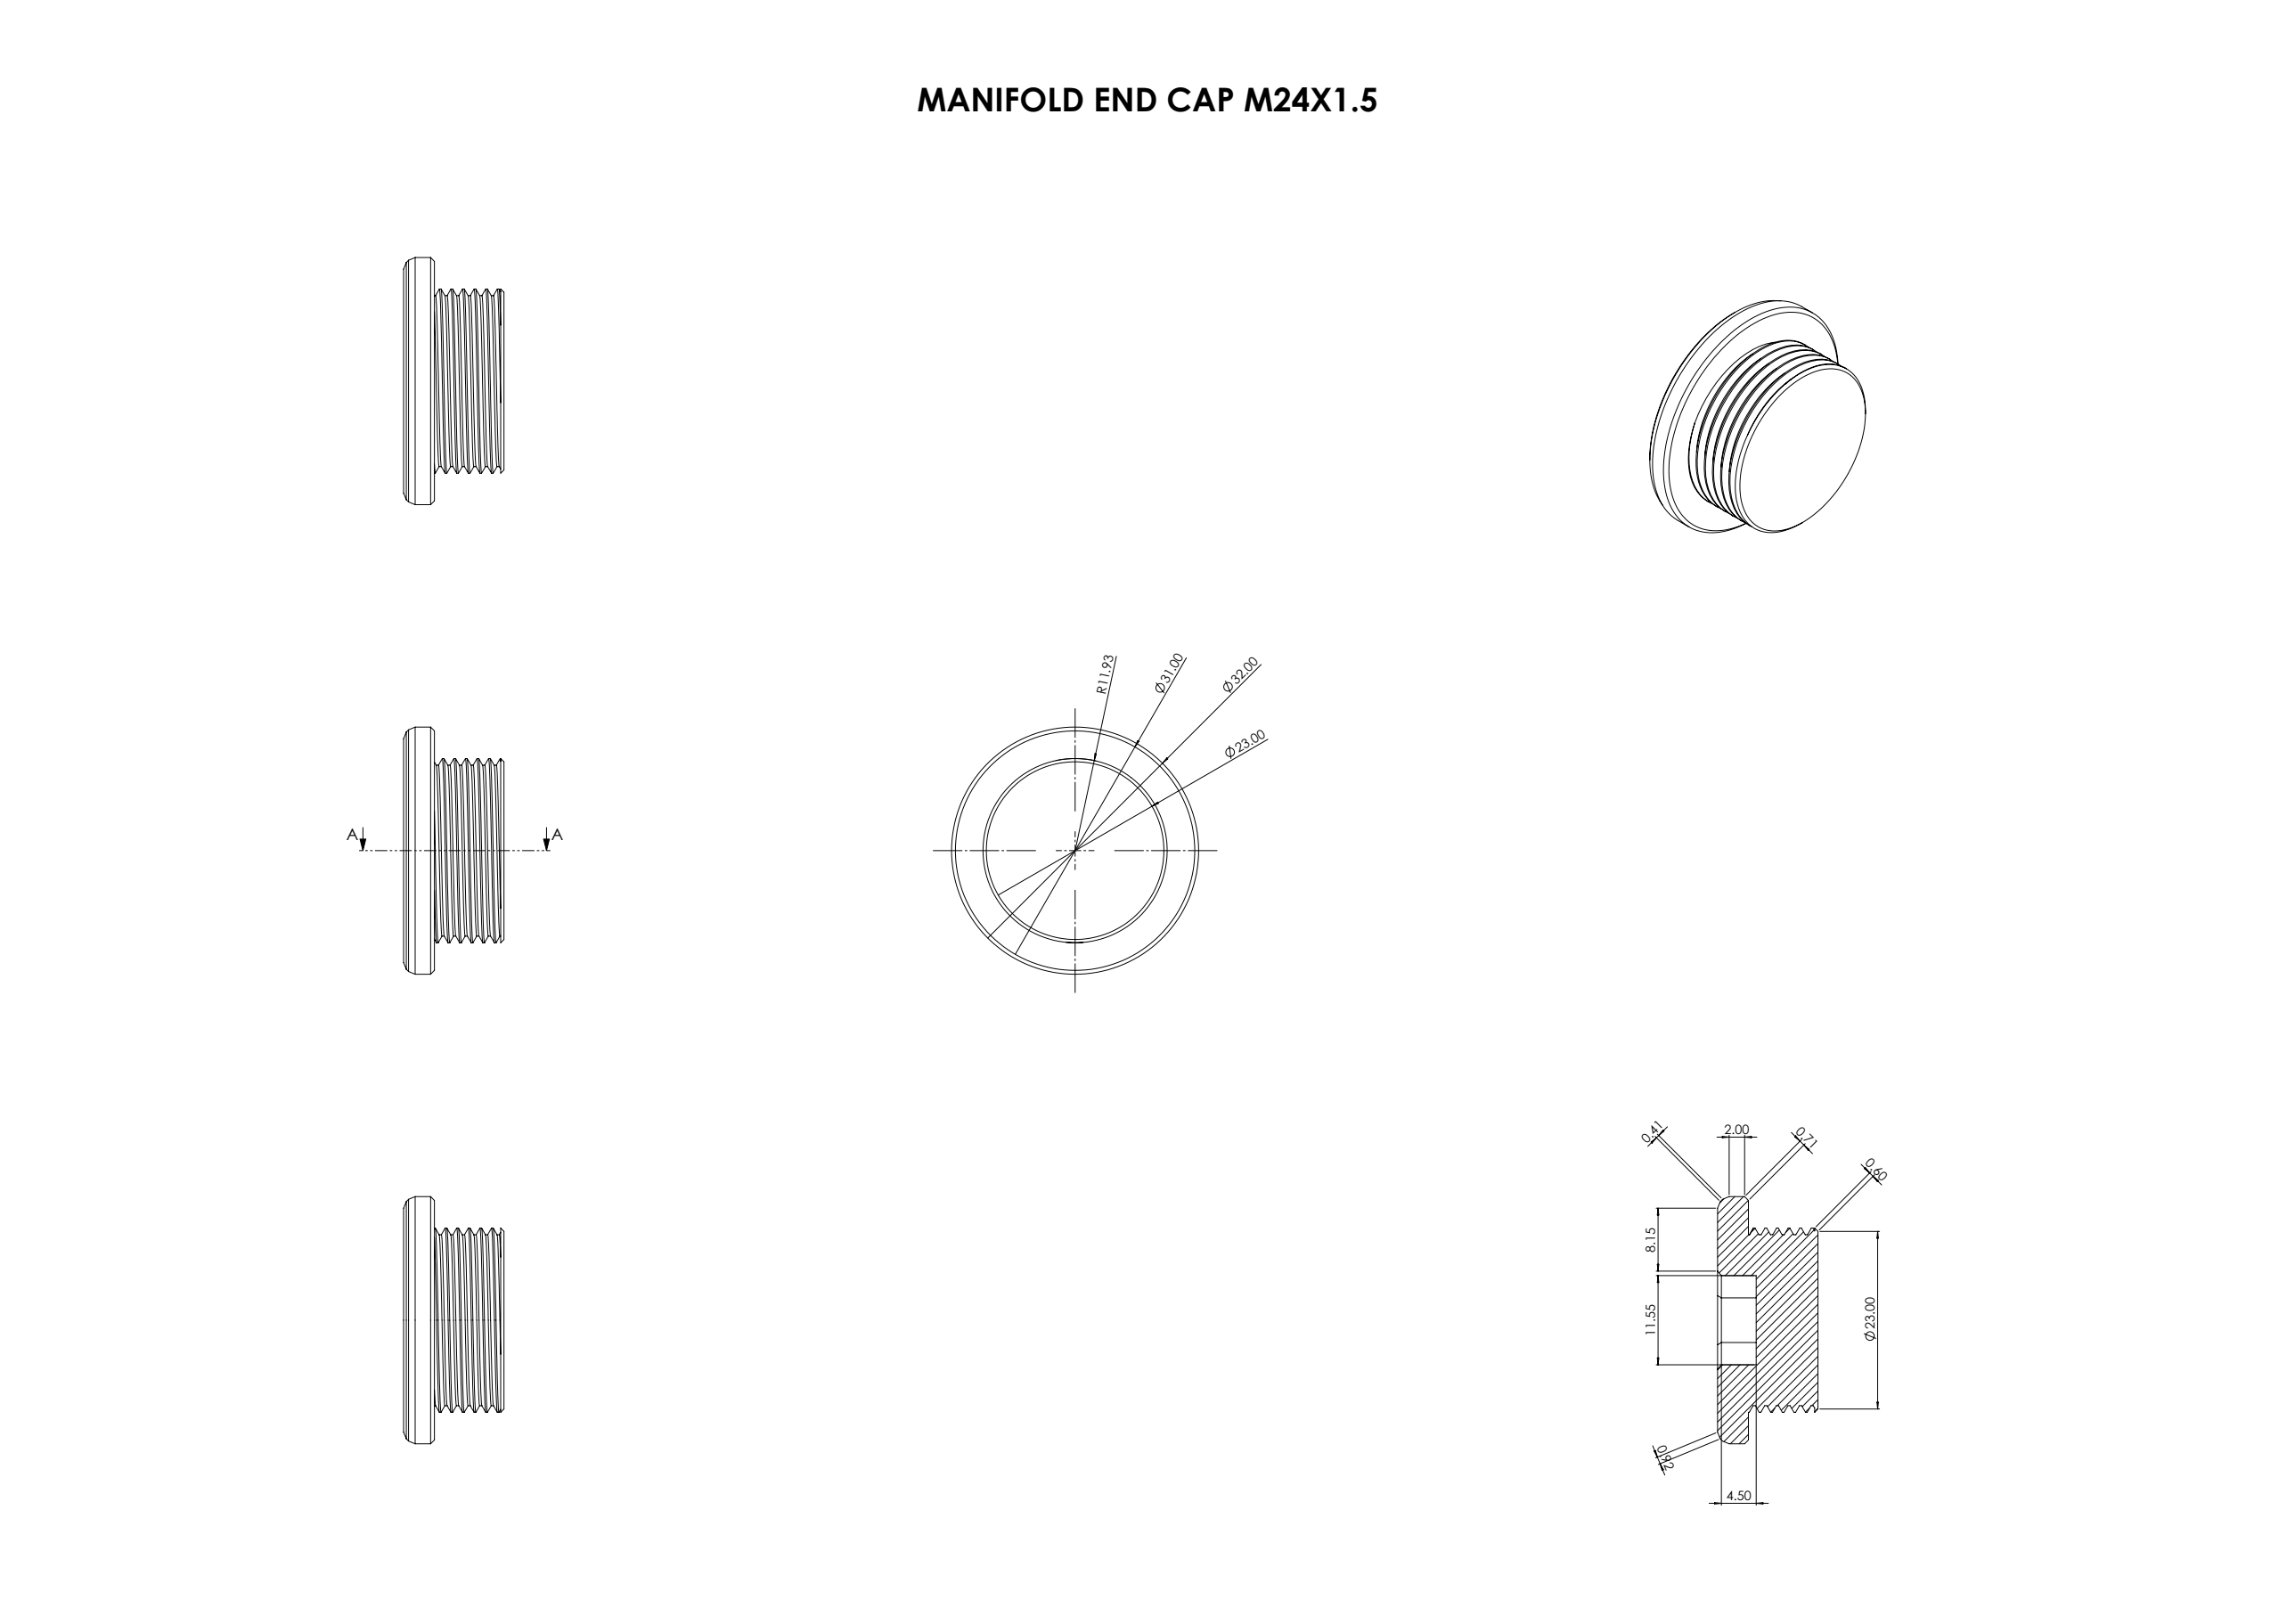
ISO-10303-21;
HEADER;
/* Generated by software containing ST-Developer
 * from STEP Tools, Inc. (www.steptools.com) 
 */

FILE_DESCRIPTION(
/* description */ (''),
/* implementation_level */ '2;1');

FILE_NAME(
/* name */ '11_Manifold_End_Cap_M24x1.5.step',
/* time_stamp */ '2026-10-26T06:13:19-07:00',
/* author */ (''),
/* organization */ (''),
/* preprocessor_version */ 'ST-DEVELOPER v20.2',
/* originating_system */ 'Autodesk Translation Framework v15.15.0.0',
/* authorisation */ '');

FILE_SCHEMA (('AUTOMOTIVE_DESIGN { 1 0 10303 214 3 1 1 }','TECHNICAL_DATA_PACKAGING'));
ENDSEC;

DATA;
#10=MECHANICAL_DESIGN_GEOMETRIC_PRESENTATION_REPRESENTATION('',(#307),#56639);
#267=SHAPE_REPRESENTATION_RELATIONSHIP('SRR','None',#56755,#287);
#287=ADVANCED_BREP_SHAPE_REPRESENTATION('',(#327),#56629);
#307=STYLED_ITEM('',(#56901),#327);
#327=MANIFOLD_SOLID_BREP('Body1',#16959);
#353=B_SPLINE_SURFACE_WITH_KNOTS('',3,3,((#35356,#35357,#35358,#35359,#35360,
#35361,#35362,#35363,#35364,#35365,#35366,#35367,#35368,#35369,#35370,#35371,
#35372,#35373,#35374,#35375,#35376,#35377,#35378,#35379,#35380,#35381,#35382,
#35383,#35384,#35385,#35386,#35387,#35388,#35389,#35390,#35391,#35392,#35393,
#35394,#35395,#35396,#35397,#35398,#35399,#35400,#35401,#35402,#35403,#35404,
#35405,#35406,#35407,#35408,#35409,#35410,#35411,#35412,#35413,#35414,#35415,
#35416,#35417,#35418,#35419,#35420,#35421,#35422,#35423,#35424,#35425,#35426,
#35427,#35428,#35429,#35430,#35431,#35432,#35433,#35434),(#35435,#35436,
#35437,#35438,#35439,#35440,#35441,#35442,#35443,#35444,#35445,#35446,#35447,
#35448,#35449,#35450,#35451,#35452,#35453,#35454,#35455,#35456,#35457,#35458,
#35459,#35460,#35461,#35462,#35463,#35464,#35465,#35466,#35467,#35468,#35469,
#35470,#35471,#35472,#35473,#35474,#35475,#35476,#35477,#35478,#35479,#35480,
#35481,#35482,#35483,#35484,#35485,#35486,#35487,#35488,#35489,#35490,#35491,
#35492,#35493,#35494,#35495,#35496,#35497,#35498,#35499,#35500,#35501,#35502,
#35503,#35504,#35505,#35506,#35507,#35508,#35509,#35510,#35511,#35512,#35513),
(#35514,#35515,#35516,#35517,#35518,#35519,#35520,#35521,#35522,#35523,
#35524,#35525,#35526,#35527,#35528,#35529,#35530,#35531,#35532,#35533,#35534,
#35535,#35536,#35537,#35538,#35539,#35540,#35541,#35542,#35543,#35544,#35545,
#35546,#35547,#35548,#35549,#35550,#35551,#35552,#35553,#35554,#35555,#35556,
#35557,#35558,#35559,#35560,#35561,#35562,#35563,#35564,#35565,#35566,#35567,
#35568,#35569,#35570,#35571,#35572,#35573,#35574,#35575,#35576,#35577,#35578,
#35579,#35580,#35581,#35582,#35583,#35584,#35585,#35586,#35587,#35588,#35589,
#35590,#35591,#35592),(#35593,#35594,#35595,#35596,#35597,#35598,#35599,
#35600,#35601,#35602,#35603,#35604,#35605,#35606,#35607,#35608,#35609,#35610,
#35611,#35612,#35613,#35614,#35615,#35616,#35617,#35618,#35619,#35620,#35621,
#35622,#35623,#35624,#35625,#35626,#35627,#35628,#35629,#35630,#35631,#35632,
#35633,#35634,#35635,#35636,#35637,#35638,#35639,#35640,#35641,#35642,#35643,
#35644,#35645,#35646,#35647,#35648,#35649,#35650,#35651,#35652,#35653,#35654,
#35655,#35656,#35657,#35658,#35659,#35660,#35661,#35662,#35663,#35664,#35665,
#35666,#35667,#35668,#35669,#35670,#35671)),.UNSPECIFIED.,.F.,.F.,.F.,(4,
4),(4,1,1,1,1,1,1,1,1,1,1,1,1,1,1,1,1,1,1,1,1,1,1,1,1,1,1,1,1,1,1,1,1,1,
1,1,1,1,1,1,1,1,1,1,1,1,1,1,1,1,1,1,1,1,1,1,1,1,1,1,1,1,1,1,1,1,1,1,1,1,
1,1,1,1,1,1,4),(0.,0.0991945497494695),(8.29865039549532,8.79860305073002,
9.29855570596471,9.79850836119941,10.2984610164341,10.7984136716688,11.2983663269035,
11.7983189821382,12.2982716373729,12.7982242926076,13.2981769478423,13.798129603077,
14.2980822583117,14.7980349135464,15.2979875687811,15.7979402240158,16.2978928792505,
16.7978455344852,17.2977981897199,17.7977508449546,18.2977035001893,18.797656155424,
19.2976088106587,19.7975614658934,20.2975141211281,20.7974667763628,21.2974194315975,
21.7973720868322,22.2973247420669,22.7972773973016,23.2972300525363,23.797182707771,
24.2971353630057,24.7970880182404,25.2970406734751,25.7969933287098,26.2969459839445,
26.7968986391792,27.2968512944139,27.7968039496486,28.2967566048833,28.796709260118,
29.2966619153527,29.7966145705874,30.2965672258221,30.7965198810568,31.2964725362915,
31.7964251915262,32.2963778467609,32.7963305019956,33.2962831572303,33.796235812465,
34.2961884676997,34.7961411229344,35.2960937781691,35.7960464334038,36.2959990886385,
36.7959517438732,37.2959043991079,37.7958570543426,38.2958097095773,38.795762364812,
39.2957150200467,39.7956676752814,40.2956203305161,40.7955729857508,41.2955256409855,
41.7954782962202,42.2954309514549,42.7953836066896,43.2953362619243,43.795288917159,
44.2952415723937,44.7951942276284,45.2951468828631,45.7950995380978,46.2950521933325),
 .UNSPECIFIED.);
#354=B_SPLINE_SURFACE_WITH_KNOTS('',3,3,((#35721,#35722,#35723,#35724,#35725,
#35726,#35727,#35728,#35729,#35730,#35731,#35732,#35733,#35734,#35735,#35736,
#35737,#35738,#35739,#35740,#35741,#35742,#35743,#35744,#35745,#35746,#35747,
#35748,#35749,#35750,#35751,#35752,#35753,#35754,#35755,#35756,#35757,#35758,
#35759,#35760,#35761,#35762,#35763,#35764,#35765,#35766,#35767,#35768,#35769,
#35770,#35771,#35772,#35773,#35774,#35775,#35776,#35777,#35778,#35779,#35780,
#35781,#35782,#35783,#35784,#35785,#35786,#35787,#35788,#35789,#35790,#35791,
#35792,#35793,#35794,#35795,#35796,#35797,#35798,#35799),(#35800,#35801,
#35802,#35803,#35804,#35805,#35806,#35807,#35808,#35809,#35810,#35811,#35812,
#35813,#35814,#35815,#35816,#35817,#35818,#35819,#35820,#35821,#35822,#35823,
#35824,#35825,#35826,#35827,#35828,#35829,#35830,#35831,#35832,#35833,#35834,
#35835,#35836,#35837,#35838,#35839,#35840,#35841,#35842,#35843,#35844,#35845,
#35846,#35847,#35848,#35849,#35850,#35851,#35852,#35853,#35854,#35855,#35856,
#35857,#35858,#35859,#35860,#35861,#35862,#35863,#35864,#35865,#35866,#35867,
#35868,#35869,#35870,#35871,#35872,#35873,#35874,#35875,#35876,#35877,#35878),
(#35879,#35880,#35881,#35882,#35883,#35884,#35885,#35886,#35887,#35888,
#35889,#35890,#35891,#35892,#35893,#35894,#35895,#35896,#35897,#35898,#35899,
#35900,#35901,#35902,#35903,#35904,#35905,#35906,#35907,#35908,#35909,#35910,
#35911,#35912,#35913,#35914,#35915,#35916,#35917,#35918,#35919,#35920,#35921,
#35922,#35923,#35924,#35925,#35926,#35927,#35928,#35929,#35930,#35931,#35932,
#35933,#35934,#35935,#35936,#35937,#35938,#35939,#35940,#35941,#35942,#35943,
#35944,#35945,#35946,#35947,#35948,#35949,#35950,#35951,#35952,#35953,#35954,
#35955,#35956,#35957),(#35958,#35959,#35960,#35961,#35962,#35963,#35964,
#35965,#35966,#35967,#35968,#35969,#35970,#35971,#35972,#35973,#35974,#35975,
#35976,#35977,#35978,#35979,#35980,#35981,#35982,#35983,#35984,#35985,#35986,
#35987,#35988,#35989,#35990,#35991,#35992,#35993,#35994,#35995,#35996,#35997,
#35998,#35999,#36000,#36001,#36002,#36003,#36004,#36005,#36006,#36007,#36008,
#36009,#36010,#36011,#36012,#36013,#36014,#36015,#36016,#36017,#36018,#36019,
#36020,#36021,#36022,#36023,#36024,#36025,#36026,#36027,#36028,#36029,#36030,
#36031,#36032,#36033,#36034,#36035,#36036)),.UNSPECIFIED.,.F.,.F.,.F.,(4,
4),(4,1,1,1,1,1,1,1,1,1,1,1,1,1,1,1,1,1,1,1,1,1,1,1,1,1,1,1,1,1,1,1,1,1,
1,1,1,1,1,1,1,1,1,1,1,1,1,1,1,1,1,1,1,1,1,1,1,1,1,1,1,1,1,1,1,1,1,1,1,1,
1,1,1,1,1,1,4),(0.,0.0991945497494695),(11.6149723878396,12.1149250430743,
12.614877698309,13.1148303535437,13.6147830087784,14.1147356640131,14.6146883192478,
15.1146409744825,15.6145936297172,16.1145462849519,16.6144989401866,17.1144515954213,
17.614404250656,18.1143569058907,18.6143095611254,19.1142622163601,19.6142148715948,
20.1141675268295,20.6141201820642,21.1140728372989,21.6140254925336,22.1139781477683,
22.613930803003,23.1138834582377,23.6138361134724,24.1137887687071,24.6137414239418,
25.1136940791765,25.6136467344112,26.1135993896459,26.6135520448806,27.1135047001153,
27.61345735535,28.1134100105847,28.6133626658194,29.1133153210541,29.6132679762888,
30.1132206315235,30.6131732867582,31.1131259419929,31.6130785972276,32.1130312524623,
32.612983907697,33.1129365629317,33.6128892181664,34.1128418734011,34.6127945286358,
35.1127471838705,35.6126998391052,36.1126524943399,36.6126051495746,37.1125578048093,
37.612510460044,38.1124631152787,38.6124157705134,39.1123684257481,39.6123210809828,
40.1122737362175,40.6122263914522,41.1121790466869,41.6121317019216,42.1120843571563,
42.612037012391,43.1119896676257,43.6119423228604,44.1118949780951,44.6118476333298,
45.1118002885645,45.6117529437992,46.1117055990339,46.6116582542686,47.1116109095033,
47.611563564738,48.1115162199727,48.6114688752074,49.1114215304421,49.6113741856768),
 .UNSPECIFIED.);
#534=FACE_BOUND('',#3333,.T.);
#535=FACE_BOUND('',#3338,.T.);
#609=CONICAL_SURFACE('',#18026,15.75,0.785398163397442);
#610=CONICAL_SURFACE('',#18035,15.8232233047034,0.392699081698714);
#611=CONICAL_SURFACE('',#18038,15.5,0.785398163397451);
#612=CONICAL_SURFACE('',#18041,14.9267766952966,1.17809724509618);
#613=CONICAL_SURFACE('',#18063,11.75,0.785398163397442);
#1057=CIRCLE('',#18012,11.925);
#1058=CIRCLE('',#18019,11.06595);
#1059=CIRCLE('',#18021,11.06595);
#1060=CIRCLE('',#18027,15.5);
#1061=CIRCLE('',#18028,16.);
#1062=CIRCLE('',#18029,16.);
#1063=CIRCLE('',#18031,16.);
#1064=CIRCLE('',#18032,16.);
#1065=CIRCLE('',#18034,11.06595);
#1066=CIRCLE('',#18036,15.6464466094067);
#1067=CIRCLE('',#18037,15.6464466094067);
#1068=CIRCLE('',#18039,15.3535533905933);
#1069=CIRCLE('',#18040,15.3535533905933);
#1070=CIRCLE('',#18042,14.5);
#1071=CIRCLE('',#18054,11.925);
#1072=CIRCLE('',#18055,11.925);
#1073=CIRCLE('',#18058,11.925);
#1074=CIRCLE('',#18064,11.5);
#1425=CYLINDRICAL_SURFACE('',#18011,11.925);
#1426=CYLINDRICAL_SURFACE('',#18013,11.925);
#1427=CYLINDRICAL_SURFACE('',#18014,11.925);
#1428=CYLINDRICAL_SURFACE('',#18015,11.925);
#1429=CYLINDRICAL_SURFACE('',#18016,11.925);
#1430=CYLINDRICAL_SURFACE('',#18017,11.925);
#1431=CYLINDRICAL_SURFACE('',#18018,11.06595);
#1432=CYLINDRICAL_SURFACE('',#18020,11.06595);
#1433=CYLINDRICAL_SURFACE('',#18022,11.06595);
#1434=CYLINDRICAL_SURFACE('',#18023,11.06595);
#1435=CYLINDRICAL_SURFACE('',#18024,11.06595);
#1436=CYLINDRICAL_SURFACE('',#18025,11.06595);
#1437=CYLINDRICAL_SURFACE('',#18030,16.);
#1438=CYLINDRICAL_SURFACE('',#18056,11.06595);
#1439=CYLINDRICAL_SURFACE('',#18057,11.925);
#2225=FACE_OUTER_BOUND('',#3318,.T.);
#2226=FACE_OUTER_BOUND('',#3319,.T.);
#2227=FACE_OUTER_BOUND('',#3320,.T.);
#2228=FACE_OUTER_BOUND('',#3321,.T.);
#2229=FACE_OUTER_BOUND('',#3322,.T.);
#2230=FACE_OUTER_BOUND('',#3323,.T.);
#2231=FACE_OUTER_BOUND('',#3324,.T.);
#2232=FACE_OUTER_BOUND('',#3325,.T.);
#2233=FACE_OUTER_BOUND('',#3326,.T.);
#2234=FACE_OUTER_BOUND('',#3327,.T.);
#2235=FACE_OUTER_BOUND('',#3328,.T.);
#2236=FACE_OUTER_BOUND('',#3329,.T.);
#2237=FACE_OUTER_BOUND('',#3330,.T.);
#2238=FACE_OUTER_BOUND('',#3331,.T.);
#2239=FACE_OUTER_BOUND('',#3332,.T.);
#2240=FACE_OUTER_BOUND('',#3334,.T.);
#2241=FACE_OUTER_BOUND('',#3335,.T.);
#2242=FACE_OUTER_BOUND('',#3336,.T.);
#2243=FACE_OUTER_BOUND('',#3337,.T.);
#2244=FACE_OUTER_BOUND('',#3339,.T.);
#2245=FACE_OUTER_BOUND('',#3340,.T.);
#2246=FACE_OUTER_BOUND('',#3341,.T.);
#2247=FACE_OUTER_BOUND('',#3342,.T.);
#2248=FACE_OUTER_BOUND('',#3343,.T.);
#2249=FACE_OUTER_BOUND('',#3344,.T.);
#2250=FACE_OUTER_BOUND('',#3345,.T.);
#2251=FACE_OUTER_BOUND('',#3346,.T.);
#2252=FACE_OUTER_BOUND('',#3347,.T.);
#2253=FACE_OUTER_BOUND('',#3348,.T.);
#2254=FACE_OUTER_BOUND('',#3349,.T.);
#2255=FACE_OUTER_BOUND('',#3350,.T.);
#2256=FACE_OUTER_BOUND('',#3351,.T.);
#2257=FACE_OUTER_BOUND('',#3352,.T.);
#2258=FACE_OUTER_BOUND('',#3353,.T.);
#2259=FACE_OUTER_BOUND('',#3354,.T.);
#2260=FACE_OUTER_BOUND('',#3355,.T.);
#2261=FACE_OUTER_BOUND('',#3356,.T.);
#2262=FACE_OUTER_BOUND('',#3357,.T.);
#2263=FACE_OUTER_BOUND('',#3358,.T.);
#3318=EDGE_LOOP('',(#12806,#12807,#12808,#12809));
#3319=EDGE_LOOP('',(#12810,#12811,#12812,#12813));
#3320=EDGE_LOOP('',(#12814,#12815,#12816,#12817));
#3321=EDGE_LOOP('',(#12818,#12819,#12820,#12821));
#3322=EDGE_LOOP('',(#12822,#12823,#12824,#12825));
#3323=EDGE_LOOP('',(#12826,#12827,#12828,#12829));
#3324=EDGE_LOOP('',(#12830,#12831,#12832));
#3325=EDGE_LOOP('',(#12833,#12834,#12835,#12836,#12837));
#3326=EDGE_LOOP('',(#12838,#12839,#12840,#12841));
#3327=EDGE_LOOP('',(#12842,#12843,#12844,#12845));
#3328=EDGE_LOOP('',(#12846,#12847,#12848,#12849));
#3329=EDGE_LOOP('',(#12850,#12851,#12852,#12853));
#3330=EDGE_LOOP('',(#12854,#12855,#12856,#12857,#12858));
#3331=EDGE_LOOP('',(#12859,#12860,#12861,#12862,#12863,#12864));
#3332=EDGE_LOOP('',(#12865));
#3333=EDGE_LOOP('',(#12866,#12867,#12868,#12869));
#3334=EDGE_LOOP('',(#12870,#12871,#12872,#12873,#12874,#12875));
#3335=EDGE_LOOP('',(#12876,#12877,#12878,#12879,#12880,#12881));
#3336=EDGE_LOOP('',(#12882,#12883,#12884,#12885,#12886));
#3337=EDGE_LOOP('',(#12887));
#3338=EDGE_LOOP('',(#12888,#12889,#12890,#12891,#12892,#12893));
#3339=EDGE_LOOP('',(#12894,#12895,#12896,#12897));
#3340=EDGE_LOOP('',(#12898,#12899,#12900,#12901));
#3341=EDGE_LOOP('',(#12902,#12903,#12904,#12905));
#3342=EDGE_LOOP('',(#12906,#12907,#12908,#12909));
#3343=EDGE_LOOP('',(#12910,#12911,#12912,#12913));
#3344=EDGE_LOOP('',(#12914,#12915,#12916,#12917));
#3345=EDGE_LOOP('',(#12918,#12919,#12920,#12921));
#3346=EDGE_LOOP('',(#12922,#12923,#12924,#12925));
#3347=EDGE_LOOP('',(#12926,#12927,#12928,#12929));
#3348=EDGE_LOOP('',(#12930,#12931,#12932,#12933,#12934,#12935));
#3349=EDGE_LOOP('',(#12936,#12937,#12938,#12939,#12940,#12941,#12942,#12943,
#12944,#12945,#12946,#12947,#12948,#12949,#12950));
#3350=EDGE_LOOP('',(#12951,#12952,#12953,#12954));
#3351=EDGE_LOOP('',(#12955,#12956,#12957,#12958,#12959,#12960,#12961,#12962,
#12963,#12964,#12965,#12966,#12967,#12968,#12969,#12970));
#3352=EDGE_LOOP('',(#12971,#12972,#12973,#12974));
#3353=EDGE_LOOP('',(#12975,#12976,#12977,#12978));
#3354=EDGE_LOOP('',(#12979,#12980,#12981,#12982));
#3355=EDGE_LOOP('',(#12983,#12984,#12985,#12986));
#3356=EDGE_LOOP('',(#12987,#12988,#12989,#12990,#12991,#12992));
#3357=EDGE_LOOP('',(#12993,#12994,#12995,#12996,#12997,#12998));
#3358=EDGE_LOOP('',(#12999));
#4255=LINE('',#34069,#5209);
#4256=LINE('',#34102,#5210);
#4257=LINE('',#34186,#5211);
#4258=LINE('',#34276,#5212);
#4259=LINE('',#34360,#5213);
#4260=LINE('',#34450,#5214);
#4261=LINE('',#34540,#5215);
#4262=LINE('',#34550,#5216);
#4263=LINE('',#34587,#5217);
#4264=LINE('',#34625,#5218);
#4265=LINE('',#34662,#5219);
#4266=LINE('',#34699,#5220);
#4267=LINE('',#34737,#5221);
#4268=LINE('',#34743,#5222);
#4269=LINE('',#35019,#5223);
#4270=LINE('',#35025,#5224);
#4271=LINE('',#35031,#5225);
#4272=LINE('',#35036,#5226);
#4273=LINE('',#35038,#5227);
#4274=LINE('',#35040,#5228);
#4275=LINE('',#35042,#5229);
#4276=LINE('',#35044,#5230);
#4277=LINE('',#35045,#5231);
#4278=LINE('',#35048,#5232);
#4279=LINE('',#35050,#5233);
#4280=LINE('',#35051,#5234);
#4281=LINE('',#35054,#5235);
#4282=LINE('',#35055,#5236);
#4283=LINE('',#35058,#5237);
#4284=LINE('',#35060,#5238);
#4285=LINE('',#35061,#5239);
#4286=LINE('',#35064,#5240);
#4287=LINE('',#35065,#5241);
#4288=LINE('',#35067,#5242);
#4289=LINE('',#35069,#5243);
#4290=LINE('',#35072,#5244);
#4291=LINE('',#35074,#5245);
#4292=LINE('',#35075,#5246);
#4293=LINE('',#35078,#5247);
#4294=LINE('',#35079,#5248);
#4295=LINE('',#35082,#5249);
#4296=LINE('',#35083,#5250);
#4297=LINE('',#36057,#5251);
#4298=LINE('',#36058,#5252);
#4299=LINE('',#36061,#5253);
#4300=LINE('',#36062,#5254);
#4301=LINE('',#36064,#5255);
#4302=LINE('',#36069,#5256);
#5209=VECTOR('',#20787,12.);
#5210=VECTOR('',#20792,12.);
#5211=VECTOR('',#20795,12.);
#5212=VECTOR('',#20798,12.);
#5213=VECTOR('',#20801,12.);
#5214=VECTOR('',#20804,12.);
#5215=VECTOR('',#20807,11.06595);
#5216=VECTOR('',#20812,11.06595);
#5217=VECTOR('',#20817,11.06595);
#5218=VECTOR('',#20820,11.06595);
#5219=VECTOR('',#20823,11.06595);
#5220=VECTOR('',#20826,11.06595);
#5221=VECTOR('',#20831,15.75);
#5222=VECTOR('',#20838,16.);
#5223=VECTOR('',#20849,15.8232233047034);
#5224=VECTOR('',#20856,15.5);
#5225=VECTOR('',#20863,14.9267766952966);
#5226=VECTOR('',#20868,10.);
#5227=VECTOR('',#20869,10.);
#5228=VECTOR('',#20870,10.);
#5229=VECTOR('',#20871,10.);
#5230=VECTOR('',#20872,10.);
#5231=VECTOR('',#20873,10.);
#5232=VECTOR('',#20876,10.);
#5233=VECTOR('',#20877,10.);
#5234=VECTOR('',#20878,10.);
#5235=VECTOR('',#20881,10.);
#5236=VECTOR('',#20882,10.);
#5237=VECTOR('',#20885,10.);
#5238=VECTOR('',#20886,10.);
#5239=VECTOR('',#20887,10.);
#5240=VECTOR('',#20890,10.);
#5241=VECTOR('',#20891,10.);
#5242=VECTOR('',#20894,10.);
#5243=VECTOR('',#20897,10.);
#5244=VECTOR('',#20900,10.);
#5245=VECTOR('',#20901,10.);
#5246=VECTOR('',#20902,10.);
#5247=VECTOR('',#20905,10.);
#5248=VECTOR('',#20906,10.);
#5249=VECTOR('',#20909,10.);
#5250=VECTOR('',#20910,10.);
#5251=VECTOR('',#20925,10.);
#5252=VECTOR('',#20926,10.);
#5253=VECTOR('',#20929,10.);
#5254=VECTOR('',#20930,10.);
#5255=VECTOR('',#20933,10.);
#5256=VECTOR('',#20940,11.75);
#6054=B_SPLINE_CURVE_WITH_KNOTS('',3,(#34071,#34072,#34073,#34074,#34075,
#34076,#34077,#34078,#34079,#34080,#34081,#34082,#34083,#34084,#34085,#34086),
 .UNSPECIFIED.,.F.,.F.,(4,3,3,3,3,4),(-4.09299088010938,-3.9996212418776,
-3.4996685866429,-2.9997159314082,-2.4997632761735,-2.07752579179387),
 .UNSPECIFIED.);
#6055=B_SPLINE_CURVE_WITH_KNOTS('',3,(#34089,#34090,#34091,#34092,#34093,
#34094,#34095,#34096,#34097,#34098),.UNSPECIFIED.,.F.,.F.,(4,3,3,4),(0.,
0.4999526552347,0.999905310469399,1.12612756527404),.UNSPECIFIED.);
#6056=B_SPLINE_CURVE_WITH_KNOTS('',3,(#34103,#34104,#34105,#34106,#34107,
#34108,#34109,#34110,#34111,#34112,#34113,#34114,#34115,#34116,#34117,#34118,
#34119,#34120,#34121,#34122,#34123,#34124,#34125,#34126,#34127,#34128,#34129,
#34130,#34131,#34132,#34133,#34134,#34135,#34136,#34137,#34138,#34139,#34140,
#34141,#34142),.UNSPECIFIED.,.F.,.F.,(4,3,3,3,3,3,3,3,3,3,3,3,3,4),(-10.376176187289,
-9.999053104694,-9.4991004494593,-8.9991477942246,-8.4991951389899,-7.9992424837552,
-7.4992898285205,-6.9993371732858,-6.4993845180511,-5.9994318628164,-5.4994792075817,
-4.999526552347,-4.4995738971123,-4.09299088010938),.UNSPECIFIED.);
#6057=B_SPLINE_CURVE_WITH_KNOTS('',3,(#34143,#34144,#34145,#34146,#34147,
#34148,#34149,#34150,#34151,#34152,#34153,#34154,#34155,#34156,#34157,#34158,
#34159,#34160,#34161,#34162,#34163,#34164,#34165,#34166,#34167,#34168,#34169,
#34170,#34171,#34172,#34173,#34174,#34175,#34176,#34177,#34178,#34179,#34180,
#34181,#34182),.UNSPECIFIED.,.F.,.F.,(4,3,3,3,3,3,3,3,3,3,3,3,3,4),(1.12612756527404,
1.4998579657041,1.9998106209388,2.4997632761735,2.9997159314082,3.4996685866429,
3.9996212418776,4.4995738971123,4.999526552347,5.4994792075817,5.9994318628164,
6.4993845180511,6.9993371732858,7.40931287245364),.UNSPECIFIED.);
#6058=B_SPLINE_CURVE_WITH_KNOTS('',3,(#34187,#34188,#34189,#34190,#34191,
#34192,#34193,#34194,#34195,#34196,#34197,#34198,#34199,#34200,#34201,#34202,
#34203,#34204,#34205,#34206,#34207,#34208,#34209,#34210,#34211,#34212,#34213,
#34214,#34215,#34216,#34217,#34218,#34219,#34220,#34221,#34222,#34223,#34224,
#34225,#34226,#34227,#34228,#34229),.UNSPECIFIED.,.F.,.F.,(4,3,3,3,3,3,
3,3,3,3,3,3,3,3,4),(-16.6593614944686,-16.4984376227451,-15.9984849675104,
-15.4985323122757,-14.998579657041,-14.4986270018063,-13.9986743465716,
-13.4987216913369,-12.9987690361022,-12.4988163808675,-11.9988637256328,
-11.4989110703981,-10.9989584151634,-10.4990057599287,-10.376176187289),
 .UNSPECIFIED.);
#6059=B_SPLINE_CURVE_WITH_KNOTS('',3,(#34230,#34231,#34232,#34233,#34234,
#34235,#34236,#34237,#34238,#34239,#34240,#34241,#34242,#34243,#34244,#34245,
#34246,#34247,#34248,#34249,#34250,#34251,#34252,#34253,#34254,#34255,#34256,
#34257,#34258,#34259,#34260,#34261,#34262,#34263,#34264,#34265,#34266,#34267,
#34268,#34269,#34270,#34271,#34272),.UNSPECIFIED.,.F.,.F.,(4,3,3,3,3,3,
3,3,3,3,3,3,3,3,4),(7.40931287245364,7.4992898285205,7.9992424837552,8.4991951389899,
8.9991477942246,9.49910044945929,9.999053104694,10.4990057599287,10.9989584151634,
11.4989110703981,11.9988637256328,12.4988163808675,12.9987690361022,13.4987216913369,
13.6924981796332),.UNSPECIFIED.);
#6060=B_SPLINE_CURVE_WITH_KNOTS('',3,(#34277,#34278,#34279,#34280,#34281,
#34282,#34283,#34284,#34285,#34286,#34287,#34288,#34289,#34290,#34291,#34292,
#34293,#34294,#34295,#34296,#34297,#34298,#34299,#34300,#34301,#34302,#34303,
#34304,#34305,#34306,#34307,#34308,#34309,#34310,#34311,#34312,#34313,#34314,
#34315,#34316),.UNSPECIFIED.,.F.,.F.,(4,3,3,3,3,3,3,3,3,3,3,3,3,4),(-22.9425468016482,
-22.4978694855615,-21.9979168303268,-21.4979641750921,-20.9980115198574,
-20.4980588646227,-19.998106209388,-19.4981535541533,-18.9982008989186,
-18.4982482436839,-17.9982955884492,-17.4983429332145,-16.9983902779798,
-16.6593614944686),.UNSPECIFIED.);
#6061=B_SPLINE_CURVE_WITH_KNOTS('',3,(#34317,#34318,#34319,#34320,#34321,
#34322,#34323,#34324,#34325,#34326,#34327,#34328,#34329,#34330,#34331,#34332,
#34333,#34334,#34335,#34336,#34337,#34338,#34339,#34340,#34341,#34342,#34343,
#34344,#34345,#34346,#34347,#34348,#34349,#34350,#34351,#34352,#34353,#34354,
#34355,#34356),.UNSPECIFIED.,.F.,.F.,(4,3,3,3,3,3,3,3,3,3,3,3,3,4),(13.6924981796332,
13.9986743465716,14.4986270018063,14.998579657041,15.4985323122757,15.9984849675104,
16.4984376227451,16.9983902779798,17.4983429332145,17.9982955884492,18.4982482436839,
18.9982008989186,19.4981535541533,19.9756834868128),.UNSPECIFIED.);
#6062=B_SPLINE_CURVE_WITH_KNOTS('',3,(#34361,#34362,#34363,#34364,#34365,
#34366,#34367,#34368,#34369,#34370,#34371,#34372,#34373,#34374,#34375,#34376,
#34377,#34378,#34379,#34380,#34381,#34382,#34383,#34384,#34385,#34386,#34387,
#34388,#34389,#34390,#34391,#34392,#34393,#34394,#34395,#34396,#34397,#34398,
#34399,#34400,#34401,#34402,#34403),.UNSPECIFIED.,.F.,.F.,(4,3,3,3,3,3,
3,3,3,3,3,3,3,3,4),(-29.2257321088278,-28.9972540036126,-28.4973013483779,
-27.9973486931432,-27.4973960379085,-26.9974433826738,-26.4974907274391,
-25.9975380722044,-25.4975854169697,-24.997632761735,-24.4976801065003,
-23.9977274512656,-23.4977747960309,-22.9978221407962,-22.9425468016482),
 .UNSPECIFIED.);
#6063=B_SPLINE_CURVE_WITH_KNOTS('',3,(#34404,#34405,#34406,#34407,#34408,
#34409,#34410,#34411,#34412,#34413,#34414,#34415,#34416,#34417,#34418,#34419,
#34420,#34421,#34422,#34423,#34424,#34425,#34426,#34427,#34428,#34429,#34430,
#34431,#34432,#34433,#34434,#34435,#34436,#34437,#34438,#34439,#34440,#34441,
#34442,#34443,#34444,#34445,#34446),.UNSPECIFIED.,.F.,.F.,(4,3,3,3,3,3,
3,3,3,3,3,3,3,3,4),(19.9756834868128,19.998106209388,20.4980588646227,20.9980115198574,
21.4979641750921,21.9979168303268,22.4978694855615,22.9978221407962,23.4977747960309,
23.9977274512656,24.4976801065003,24.997632761735,25.4975854169697,25.9975380722044,
26.2588687939924),.UNSPECIFIED.);
#6064=B_SPLINE_CURVE_WITH_KNOTS('',3,(#34451,#34452,#34453,#34454,#34455,
#34456,#34457,#34458,#34459,#34460,#34461,#34462,#34463,#34464,#34465,#34466,
#34467,#34468,#34469,#34470,#34471,#34472,#34473,#34474,#34475,#34476,#34477,
#34478,#34479,#34480,#34481,#34482,#34483,#34484,#34485,#34486,#34487,#34488,
#34489,#34490,#34491,#34492,#34493),.UNSPECIFIED.,.F.,.F.,(4,3,3,3,3,3,
3,3,3,3,3,3,3,3,4),(-35.5089174160073,-35.4966385216637,-34.996685866429,
-34.4967332111943,-33.9967805559596,-33.4968279007249,-32.9968752454902,
-32.4969225902555,-31.9969699350208,-31.4970172797861,-30.9970646245514,
-30.4971119693167,-29.997159314082,-29.4972066588473,-29.2257321088278),
 .UNSPECIFIED.);
#6065=B_SPLINE_CURVE_WITH_KNOTS('',3,(#34494,#34495,#34496,#34497,#34498,
#34499,#34500,#34501,#34502,#34503,#34504,#34505,#34506,#34507,#34508,#34509,
#34510,#34511,#34512,#34513,#34514,#34515,#34516,#34517,#34518,#34519,#34520,
#34521,#34522,#34523,#34524,#34525,#34526,#34527,#34528,#34529,#34530,#34531,
#34532,#34533,#34534,#34535,#34536),.UNSPECIFIED.,.F.,.F.,(4,3,3,3,3,3,
3,3,3,3,3,3,3,3,4),(26.2588687939924,26.4974907274391,26.9974433826738,
27.4973960379085,27.9973486931432,28.4973013483779,28.9972540036126,29.4972066588473,
29.997159314082,30.4971119693167,30.9970646245514,31.4970172797861,31.9969699350208,
32.4969225902555,32.542054101172),.UNSPECIFIED.);
#6066=B_SPLINE_CURVE_WITH_KNOTS('',3,(#34542,#34543,#34544,#34545),
 .UNSPECIFIED.,.F.,.F.,(4,4),(47.1238898038469,47.5338483938829),
 .UNSPECIFIED.);
#6067=B_SPLINE_CURVE_WITH_KNOTS('',3,(#34551,#34552,#34553,#34554,#34555,
#34556,#34557,#34558,#34559,#34560,#34561,#34562,#34563,#34564,#34565,#34566,
#34567),.UNSPECIFIED.,.F.,.F.,(4,1,1,1,1,1,1,1,1,1,1,1,1,1,4),(40.8407044966673,
41.1121790466869,41.6121317019216,42.1120843571563,42.612037012391,43.1119896676257,
43.6119423228604,44.1118949780951,44.6118476333298,45.1118002885645,45.6117529437992,
46.1117055990339,46.6116582542686,47.1116109095033,47.1238898038469),
 .UNSPECIFIED.);
#6068=B_SPLINE_CURVE_WITH_KNOTS('',3,(#34570,#34571,#34572,#34573,#34574,
#34575,#34576,#34577,#34578,#34579,#34580,#34581,#34582,#34583),
 .UNSPECIFIED.,.F.,.F.,(4,1,1,1,1,1,1,1,1,1,1,4),(40.8407044966673,41.2955256409855,
41.7954782962202,42.2954309514549,42.7953836066896,43.2953362619243,43.795288917159,
44.2952415723937,44.7951942276284,45.2951468828631,45.7950995380978,46.2950521933325),
 .UNSPECIFIED.);
#6069=B_SPLINE_CURVE_WITH_KNOTS('',3,(#34588,#34589,#34590,#34591,#34592,
#34593,#34594,#34595,#34596,#34597,#34598,#34599,#34600,#34601,#34602,#34603,
#34604),.UNSPECIFIED.,.F.,.F.,(4,1,1,1,1,1,1,1,1,1,1,1,1,1,4),(34.5575191894877,
34.6127945286358,35.1127471838705,35.6126998391052,36.1126524943399,36.6126051495746,
37.1125578048093,37.612510460044,38.1124631152787,38.6124157705134,39.1123684257481,
39.6123210809828,40.1122737362175,40.6122263914522,40.8407044966673),
 .UNSPECIFIED.);
#6070=B_SPLINE_CURVE_WITH_KNOTS('',3,(#34605,#34606,#34607,#34608,#34609,
#34610,#34611,#34612,#34613,#34614,#34615,#34616,#34617,#34618,#34619,#34620,
#34621),.UNSPECIFIED.,.F.,.F.,(4,1,1,1,1,1,1,1,1,1,1,1,1,1,4),(34.5575191894877,
34.7961411229344,35.2960937781691,35.7960464334038,36.2959990886385,36.7959517438732,
37.2959043991079,37.7958570543426,38.2958097095773,38.795762364812,39.2957150200467,
39.7956676752814,40.2956203305161,40.7955729857508,40.8407044966673),
 .UNSPECIFIED.);
#6071=B_SPLINE_CURVE_WITH_KNOTS('',3,(#34626,#34627,#34628,#34629,#34630,
#34631,#34632,#34633,#34634,#34635,#34636,#34637,#34638,#34639,#34640,#34641),
 .UNSPECIFIED.,.F.,.F.,(4,1,1,1,1,1,1,1,1,1,1,1,1,4),(28.2743338823081,
28.6133626658194,29.1133153210541,29.6132679762888,30.1132206315235,30.6131732867582,
31.1131259419929,31.6130785972276,32.1130312524623,32.612983907697,33.1129365629317,
33.6128892181664,34.1128418734011,34.5575191894877),.UNSPECIFIED.);
#6072=B_SPLINE_CURVE_WITH_KNOTS('',3,(#34642,#34643,#34644,#34645,#34646,
#34647,#34648,#34649,#34650,#34651,#34652,#34653,#34654,#34655,#34656,#34657,
#34658),.UNSPECIFIED.,.F.,.F.,(4,1,1,1,1,1,1,1,1,1,1,1,1,1,4),(28.2743338823082,
28.2967566048833,28.796709260118,29.2966619153527,29.7966145705874,30.2965672258221,
30.7965198810568,31.2964725362915,31.7964251915262,32.2963778467609,32.7963305019956,
33.2962831572303,33.796235812465,34.2961884676997,34.5575191894877),
 .UNSPECIFIED.);
#6073=B_SPLINE_CURVE_WITH_KNOTS('',3,(#34663,#34664,#34665,#34666,#34667,
#34668,#34669,#34670,#34671,#34672,#34673,#34674,#34675,#34676,#34677,#34678,
#34679),.UNSPECIFIED.,.F.,.F.,(4,1,1,1,1,1,1,1,1,1,1,1,1,1,4),(21.9911485751286,
22.1139781477683,22.613930803003,23.1138834582377,23.6138361134724,24.1137887687071,
24.6137414239418,25.1136940791765,25.6136467344112,26.1135993896459,26.6135520448806,
27.1135047001153,27.61345735535,28.1134100105847,28.2743338823081),
 .UNSPECIFIED.);
#6074=B_SPLINE_CURVE_WITH_KNOTS('',3,(#34680,#34681,#34682,#34683,#34684,
#34685,#34686,#34687,#34688,#34689,#34690,#34691,#34692,#34693,#34694,#34695),
 .UNSPECIFIED.,.F.,.F.,(4,1,1,1,1,1,1,1,1,1,1,1,1,4),(21.9911485751286,
22.2973247420669,22.7972773973016,23.2972300525363,23.797182707771,24.2971353630057,
24.7970880182404,25.2970406734751,25.7969933287098,26.2969459839445,26.7968986391792,
27.2968512944139,27.7968039496486,28.2743338823082),.UNSPECIFIED.);
#6075=B_SPLINE_CURVE_WITH_KNOTS('',3,(#34700,#34701,#34702,#34703,#34704,
#34705,#34706,#34707,#34708,#34709,#34710,#34711,#34712,#34713,#34714,#34715),
 .UNSPECIFIED.,.F.,.F.,(4,1,1,1,1,1,1,1,1,1,1,1,1,4),(15.707963267949,16.1145462849519,
16.6144989401866,17.1144515954213,17.614404250656,18.1143569058907,18.6143095611254,
19.1142622163601,19.6142148715948,20.1141675268295,20.6141201820642,21.1140728372989,
21.6140254925336,21.9911485751286),.UNSPECIFIED.);
#6076=B_SPLINE_CURVE_WITH_KNOTS('',3,(#34716,#34717,#34718,#34719,#34720,
#34721,#34722,#34723,#34724,#34725,#34726,#34727,#34728,#34729,#34730,#34731,
#34732),.UNSPECIFIED.,.F.,.F.,(4,1,1,1,1,1,1,1,1,1,1,1,1,1,4),(15.707963267949,
15.7979402240158,16.2978928792505,16.7978455344852,17.2977981897199,17.7977508449546,
18.2977035001893,18.797656155424,19.2976088106587,19.7975614658934,20.2975141211281,
20.7974667763628,21.2974194315975,21.7973720868322,21.9911485751286),
 .UNSPECIFIED.);
#6077=B_SPLINE_CURVE_WITH_KNOTS('',3,(#34749,#34750,#34751,#34752,#34753,
#34754,#34755,#34756,#34757,#34758,#34759,#34760,#34761,#34762,#34763,#34764,
#34765,#34766,#34767,#34768,#34769,#34770,#34771,#34772,#34773,#34774,#34775,
#34776,#34777,#34778,#34779,#34780,#34781,#34782,#34783,#34784,#34785,#34786,
#34787,#34788,#34789,#34790,#34791,#34792,#34793,#34794,#34795,#34796,#34797,
#34798,#34799,#34800,#34801,#34802,#34803,#34804,#34805,#34806,#34807,#34808,
#34809,#34810,#34811,#34812,#34813,#34814,#34815,#34816,#34817,#34818,#34819,
#34820,#34821,#34822,#34823,#34824,#34825,#34826,#34827,#34828,#34829,#34830,
#34831,#34832,#34833,#34834,#34835,#34836,#34837,#34838,#34839,#34840,#34841,
#34842,#34843,#34844,#34845,#34846,#34847,#34848,#34849,#34850,#34851,#34852,
#34853,#34854,#34855,#34856,#34857,#34858,#34859,#34860,#34861,#34862,#34863,
#34864,#34865,#34866,#34867,#34868,#34869,#34870,#34871,#34872,#34873,#34874,
#34875,#34876,#34877,#34878,#34879,#34880,#34881),.UNSPECIFIED.,.F.,.F.,
(4,3,3,3,3,3,3,3,3,3,3,3,3,3,3,3,3,3,3,3,3,3,3,3,3,3,3,3,3,3,3,3,3,3,3,
3,3,3,3,3,3,3,3,3,4),(-2.39439908413783,-2.30957006706654,-2.30182447788038,
-2.21683915448865,-2.13179789072762,-2.10408753243577,-2.08510252693198,
-2.07378115843186,-1.9893556355058,-1.90508589622026,-1.8214508359809,-1.79406927604186,
-1.78088810955347,-1.77088744261425,-1.71192459622473,-1.62862729255915,
-1.54477045309122,-1.46093260268497,-1.37847744264543,-1.3475567576306,
-1.32641194433753,-1.31774824536313,-1.23483340159521,-1.15208726906264,
-1.13111196252681,-1.04809579862442,-0.965185364599438,-0.914579669022902,
-0.892439677208167,-0.877969102190866,-0.870243944296804,-0.788175403641409,
-0.706044208898441,-0.624661556162812,-0.56033979998715,-0.490297324988757,
-0.459653742176959,-0.439904400552519,-0.429071911295872,-0.348385668380925,
-0.267119040059977,-0.186022607101873,-0.105553521737276,-0.0264973312222494,
0.),.UNSPECIFIED.);
#6078=B_SPLINE_CURVE_WITH_KNOTS('',3,(#34884,#34885,#34886,#34887,#34888,
#34889,#34890,#34891,#34892,#34893,#34894,#34895,#34896,#34897,#34898,#34899,
#34900,#34901,#34902,#34903,#34904,#34905,#34906,#34907,#34908,#34909,#34910,
#34911,#34912,#34913,#34914,#34915,#34916,#34917,#34918,#34919,#34920,#34921,
#34922,#34923,#34924,#34925,#34926,#34927,#34928,#34929,#34930,#34931,#34932,
#34933,#34934,#34935,#34936,#34937,#34938,#34939,#34940,#34941,#34942,#34943,
#34944,#34945,#34946,#34947,#34948,#34949,#34950,#34951,#34952,#34953,#34954,
#34955,#34956,#34957,#34958,#34959,#34960,#34961,#34962,#34963,#34964,#34965,
#34966,#34967,#34968,#34969,#34970,#34971,#34972,#34973,#34974,#34975,#34976,
#34977,#34978,#34979,#34980,#34981,#34982,#34983,#34984,#34985,#34986,#34987,
#34988,#34989,#34990,#34991,#34992,#34993,#34994,#34995,#34996,#34997,#34998,
#34999,#35000,#35001,#35002,#35003,#35004,#35005,#35006,#35007,#35008,#35009,
#35010,#35011,#35012,#35013,#35014,#35015,#35016),.UNSPECIFIED.,.F.,.F.,
(4,3,3,3,3,3,3,3,3,3,3,3,3,3,3,3,3,3,3,3,3,3,3,3,3,3,3,3,3,3,3,3,3,3,3,
3,3,3,3,3,3,3,3,3,4),(-2.39814946016211,-2.31696654854078,-2.31176064552941,
-2.2311333678253,-2.15001222659785,-2.12500103373431,-2.11084475967138,
-2.10007493179954,-2.01881508560754,-1.93699475602997,-1.85542103054389,
-1.82902405810322,-1.81445850161468,-1.80514353455762,-1.7498331407812,
-1.66857359850511,-1.58641199849619,-1.50382302505166,-1.42203537088144,
-1.39136500056761,-1.37149659188763,-1.36296522535554,-1.27990647763488,
-1.19645107967923,-1.17667240837077,-1.09362128325192,-1.01021569736535,
-0.958095766843359,-0.935293297239988,-0.920835977756462,-0.912266009922214,
-0.828465696793338,-0.744201354938751,-0.660092638546984,-0.593256253189411,
-0.519099221540735,-0.486655520194439,-0.46739399444203,-0.456346246303998,
-0.372642943242295,-0.287971923540297,-0.202778852160483,-0.117861506263224,
-0.0340642945208537,0.),.UNSPECIFIED.);
#6079=B_SPLINE_CURVE_WITH_KNOTS('',3,(#35086,#35087,#35088,#35089,#35090,
#35091,#35092,#35093,#35094,#35095,#35096,#35097,#35098,#35099,#35100,#35101,
#35102,#35103,#35104,#35105,#35106,#35107,#35108,#35109,#35110,#35111,#35112,
#35113,#35114,#35115,#35116,#35117,#35118,#35119,#35120,#35121,#35122,#35123,
#35124,#35125,#35126,#35127,#35128,#35129,#35130,#35131,#35132,#35133,#35134,
#35135,#35136,#35137,#35138,#35139,#35140,#35141,#35142,#35143,#35144,#35145,
#35146,#35147,#35148,#35149,#35150,#35151,#35152,#35153,#35154,#35155,#35156,
#35157,#35158,#35159,#35160,#35161,#35162,#35163,#35164,#35165,#35166,#35167,
#35168,#35169,#35170,#35171,#35172,#35173,#35174,#35175,#35176,#35177,#35178,
#35179,#35180,#35181,#35182,#35183,#35184,#35185,#35186,#35187,#35188,#35189,
#35190,#35191,#35192,#35193,#35194,#35195,#35196,#35197,#35198,#35199,#35200,
#35201,#35202,#35203,#35204,#35205,#35206,#35207,#35208,#35209,#35210,#35211,
#35212,#35213,#35214,#35215,#35216,#35217,#35218),.UNSPECIFIED.,.F.,.F.,
(4,3,3,3,3,3,3,3,3,3,3,3,3,3,3,3,3,3,3,3,3,3,3,3,3,3,3,3,3,3,3,3,3,3,3,
3,3,3,3,3,3,3,3,3,4),(-2.39814946016209,-2.31696654798685,-2.31176064552942,
-2.23113336581782,-2.15001222437096,-2.1250010316466,-2.11084475490401,
-2.10007493009901,-2.01881508213026,-1.93699475310395,-1.85542102865954,
-1.82902405668996,-1.81445849842888,-1.80514353011277,-1.74983314078119,
-1.66857360092947,-1.58641200157897,-1.50382302878938,-1.42203537368473,
-1.39136500302049,-1.37149659340416,-1.36296522675857,-1.27990647947373,
-1.19645108306756,-1.17667240837078,-1.09362128874921,-1.01021570226622,
-0.958095771131617,-0.935293301260229,-0.92083598151022,-0.912266014498421,
-0.828465707020358,-0.744201365768398,-0.660092636593609,-0.593256253189404,
-0.519099221540729,-0.486655520194433,-0.467393994895198,-0.456346246608538,
-0.372642917004424,-0.287971879301221,-0.202778810971215,-0.117861482515254,
-0.0340643074044279,0.),.UNSPECIFIED.);
#6080=B_SPLINE_CURVE_WITH_KNOTS('',3,(#35223,#35224,#35225,#35226,#35227,
#35228,#35229,#35230,#35231,#35232,#35233,#35234,#35235,#35236,#35237,#35238,
#35239,#35240,#35241,#35242,#35243,#35244,#35245,#35246,#35247,#35248,#35249,
#35250,#35251,#35252,#35253,#35254,#35255,#35256,#35257,#35258,#35259,#35260,
#35261,#35262,#35263,#35264,#35265,#35266,#35267,#35268,#35269,#35270,#35271,
#35272,#35273,#35274,#35275,#35276,#35277,#35278,#35279,#35280,#35281,#35282,
#35283,#35284,#35285,#35286,#35287,#35288,#35289,#35290,#35291,#35292,#35293,
#35294,#35295,#35296,#35297,#35298,#35299,#35300,#35301,#35302,#35303,#35304,
#35305,#35306,#35307,#35308,#35309,#35310,#35311,#35312,#35313,#35314,#35315,
#35316,#35317,#35318,#35319,#35320,#35321,#35322,#35323,#35324,#35325,#35326,
#35327,#35328,#35329,#35330,#35331,#35332,#35333,#35334,#35335,#35336,#35337,
#35338,#35339,#35340,#35341,#35342,#35343,#35344,#35345,#35346,#35347,#35348,
#35349,#35350,#35351,#35352,#35353,#35354,#35355),.UNSPECIFIED.,.F.,.F.,
(4,3,3,3,3,3,3,3,3,3,3,3,3,3,3,3,3,3,3,3,3,3,3,3,3,3,3,3,3,3,3,3,3,3,3,
3,3,3,3,3,3,3,3,3,4),(-2.39439908413779,-2.3095700684437,-2.30182447788042,
-2.21683915479781,-2.1317978905798,-2.10408753251614,-2.08510252752977,
-2.07378115868177,-1.9893556358529,-1.90508589613195,-1.82145083606717,
-1.79406927610656,-1.78088810966333,-1.77088744287616,-1.71192459622475,
-1.62862729253653,-1.54477045235636,-1.46093259841181,-1.37847743944056,
-1.34755675482634,-1.32641194414506,-1.31774824508864,-1.2348333999042,
-1.15208726165353,-1.13111196252682,-1.04809579835495,-0.965185374476776,
-0.914579677665573,-0.892439685310672,-0.877969115241355,-0.870243964987608,
-0.788175424134281,-0.706044237682933,-0.624661608660605,-0.560339799987152,
-0.490297324988758,-0.459653742176961,-0.439904400316136,-0.429071911044687,
-0.348385687679688,-0.267119065290005,-0.186022614582263,-0.105553499032249,
-0.0264972650708247,0.),.UNSPECIFIED.);
#6081=B_SPLINE_CURVE_WITH_KNOTS('',3,(#35672,#35673,#35674,#35675,#35676,
#35677,#35678,#35679,#35680,#35681,#35682,#35683,#35684,#35685,#35686,#35687,
#35688,#35689,#35690,#35691,#35692,#35693),.UNSPECIFIED.,.F.,.F.,(4,3,3,
3,3,3,3,4),(32.542054101172,32.9968752454902,33.4968279007249,33.9967805559596,
34.4967332111943,34.996685866429,35.4966385216637,35.9188760060433),
 .UNSPECIFIED.);
#6082=B_SPLINE_CURVE_WITH_KNOTS('',3,(#35694,#35695,#35696,#35697,#35698,
#35699,#35700,#35701,#35702,#35703,#35704,#35705,#35706,#35707),
 .UNSPECIFIED.,.F.,.F.,(4,1,1,1,1,1,1,1,1,1,1,4),(10.3761761872892,10.7984136716688,
11.2983663269035,11.7983189821382,12.2982716373729,12.7982242926076,13.2981769478423,
13.798129603077,14.2980822583117,14.7980349135464,15.2979875687811,15.707963267949),
 .UNSPECIFIED.);
#6083=B_SPLINE_CURVE_WITH_KNOTS('',3,(#35709,#35710,#35711,#35712,#35713,
#35714,#35715,#35716,#35717,#35718,#35719,#35720),.UNSPECIFIED.,.F.,.F.,
(4,1,1,1,1,1,1,1,1,4),(11.6149723878396,12.1149250430743,12.614877698309,
13.1148303535437,13.6147830087784,14.1147356640131,14.6146883192478,15.1146409744825,
15.6145936297172,15.707963267949),.UNSPECIFIED.);
#6084=B_SPLINE_CURVE_WITH_KNOTS('',3,(#36037,#36038,#36039,#36040,#36041,
#36042,#36043,#36044,#36045,#36046,#36047,#36048,#36049,#36050,#36051,#36052),
 .UNSPECIFIED.,.F.,.F.,(4,3,3,3,3,4),(-37.9964017978372,-37.4964491426025,
-36.9964964873678,-36.4965438321331,-35.9965911768984,-35.5089174160073),
 .UNSPECIFIED.);
#7354=VERTEX_POINT('',#34067);
#7355=VERTEX_POINT('',#34068);
#7356=VERTEX_POINT('',#34070);
#7357=VERTEX_POINT('',#34087);
#7358=VERTEX_POINT('',#34100);
#7359=VERTEX_POINT('',#34101);
#7360=VERTEX_POINT('',#34184);
#7361=VERTEX_POINT('',#34185);
#7362=VERTEX_POINT('',#34274);
#7363=VERTEX_POINT('',#34275);
#7364=VERTEX_POINT('',#34358);
#7365=VERTEX_POINT('',#34359);
#7366=VERTEX_POINT('',#34448);
#7367=VERTEX_POINT('',#34449);
#7368=VERTEX_POINT('',#34538);
#7369=VERTEX_POINT('',#34539);
#7370=VERTEX_POINT('',#34541);
#7371=VERTEX_POINT('',#34548);
#7372=VERTEX_POINT('',#34549);
#7373=VERTEX_POINT('',#34568);
#7374=VERTEX_POINT('',#34585);
#7375=VERTEX_POINT('',#34586);
#7376=VERTEX_POINT('',#34623);
#7377=VERTEX_POINT('',#34624);
#7378=VERTEX_POINT('',#34660);
#7379=VERTEX_POINT('',#34661);
#7380=VERTEX_POINT('',#34697);
#7381=VERTEX_POINT('',#34698);
#7382=VERTEX_POINT('',#34734);
#7383=VERTEX_POINT('',#34736);
#7384=VERTEX_POINT('',#34738);
#7385=VERTEX_POINT('',#34742);
#7386=VERTEX_POINT('',#34744);
#7387=VERTEX_POINT('',#34748);
#7388=VERTEX_POINT('',#34882);
#7389=VERTEX_POINT('',#35018);
#7390=VERTEX_POINT('',#35020);
#7391=VERTEX_POINT('',#35024);
#7392=VERTEX_POINT('',#35026);
#7393=VERTEX_POINT('',#35030);
#7394=VERTEX_POINT('',#35034);
#7395=VERTEX_POINT('',#35035);
#7396=VERTEX_POINT('',#35037);
#7397=VERTEX_POINT('',#35039);
#7398=VERTEX_POINT('',#35041);
#7399=VERTEX_POINT('',#35043);
#7400=VERTEX_POINT('',#35047);
#7401=VERTEX_POINT('',#35049);
#7402=VERTEX_POINT('',#35053);
#7403=VERTEX_POINT('',#35057);
#7404=VERTEX_POINT('',#35059);
#7405=VERTEX_POINT('',#35063);
#7406=VERTEX_POINT('',#35071);
#7407=VERTEX_POINT('',#35073);
#7408=VERTEX_POINT('',#35077);
#7409=VERTEX_POINT('',#35081);
#7410=VERTEX_POINT('',#35085);
#7411=VERTEX_POINT('',#35219);
#7412=VERTEX_POINT('',#35221);
#7413=VERTEX_POINT('',#36056);
#7414=VERTEX_POINT('',#36060);
#7415=VERTEX_POINT('',#36067);
#9310=EDGE_CURVE('',#7354,#7355,#4255,.T.);
#9311=EDGE_CURVE('',#7354,#7356,#6054,.T.);
#9312=EDGE_CURVE('',#7356,#7357,#1057,.F.);
#9313=EDGE_CURVE('',#7357,#7355,#6055,.T.);
#9314=EDGE_CURVE('',#7358,#7359,#4256,.T.);
#9315=EDGE_CURVE('',#7358,#7354,#6056,.T.);
#9316=EDGE_CURVE('',#7355,#7359,#6057,.T.);
#9317=EDGE_CURVE('',#7360,#7361,#4257,.T.);
#9318=EDGE_CURVE('',#7360,#7358,#6058,.T.);
#9319=EDGE_CURVE('',#7359,#7361,#6059,.T.);
#9320=EDGE_CURVE('',#7362,#7363,#4258,.T.);
#9321=EDGE_CURVE('',#7362,#7360,#6060,.T.);
#9322=EDGE_CURVE('',#7361,#7363,#6061,.T.);
#9323=EDGE_CURVE('',#7364,#7365,#4259,.T.);
#9324=EDGE_CURVE('',#7364,#7362,#6062,.T.);
#9325=EDGE_CURVE('',#7363,#7365,#6063,.T.);
#9326=EDGE_CURVE('',#7366,#7367,#4260,.T.);
#9327=EDGE_CURVE('',#7366,#7364,#6064,.T.);
#9328=EDGE_CURVE('',#7365,#7367,#6065,.T.);
#9329=EDGE_CURVE('',#7368,#7369,#4261,.T.);
#9330=EDGE_CURVE('',#7368,#7370,#6066,.T.);
#9331=EDGE_CURVE('',#7369,#7370,#1058,.T.);
#9332=EDGE_CURVE('',#7371,#7372,#4262,.T.);
#9333=EDGE_CURVE('',#7371,#7368,#6067,.T.);
#9334=EDGE_CURVE('',#7373,#7369,#1059,.T.);
#9335=EDGE_CURVE('',#7372,#7373,#6068,.T.);
#9336=EDGE_CURVE('',#7374,#7375,#4263,.T.);
#9337=EDGE_CURVE('',#7374,#7371,#6069,.T.);
#9338=EDGE_CURVE('',#7375,#7372,#6070,.T.);
#9339=EDGE_CURVE('',#7376,#7377,#4264,.T.);
#9340=EDGE_CURVE('',#7376,#7374,#6071,.T.);
#9341=EDGE_CURVE('',#7377,#7375,#6072,.T.);
#9342=EDGE_CURVE('',#7378,#7379,#4265,.T.);
#9343=EDGE_CURVE('',#7378,#7376,#6073,.T.);
#9344=EDGE_CURVE('',#7379,#7377,#6074,.T.);
#9345=EDGE_CURVE('',#7380,#7381,#4266,.T.);
#9346=EDGE_CURVE('',#7380,#7378,#6075,.T.);
#9347=EDGE_CURVE('',#7381,#7379,#6076,.T.);
#9348=EDGE_CURVE('',#7382,#7382,#1060,.T.);
#9349=EDGE_CURVE('',#7382,#7383,#4267,.T.);
#9350=EDGE_CURVE('',#7383,#7384,#1061,.T.);
#9351=EDGE_CURVE('',#7384,#7383,#1062,.T.);
#9352=EDGE_CURVE('',#7384,#7385,#4268,.T.);
#9353=EDGE_CURVE('',#7386,#7385,#1063,.T.);
#9354=EDGE_CURVE('',#7385,#7386,#1064,.T.);
#9355=EDGE_CURVE('',#7356,#7387,#6077,.T.);
#9356=EDGE_CURVE('',#7387,#7388,#1065,.T.);
#9357=EDGE_CURVE('',#7388,#7357,#6078,.T.);
#9358=EDGE_CURVE('',#7386,#7389,#4269,.T.);
#9359=EDGE_CURVE('',#7389,#7390,#1066,.T.);
#9360=EDGE_CURVE('',#7390,#7389,#1067,.T.);
#9361=EDGE_CURVE('',#7390,#7391,#4270,.T.);
#9362=EDGE_CURVE('',#7392,#7391,#1068,.T.);
#9363=EDGE_CURVE('',#7391,#7392,#1069,.T.);
#9364=EDGE_CURVE('',#7392,#7393,#4271,.T.);
#9365=EDGE_CURVE('',#7393,#7393,#1070,.T.);
#9366=EDGE_CURVE('',#7394,#7395,#4272,.T.);
#9367=EDGE_CURVE('',#7396,#7394,#4273,.T.);
#9368=EDGE_CURVE('',#7397,#7396,#4274,.T.);
#9369=EDGE_CURVE('',#7398,#7397,#4275,.T.);
#9370=EDGE_CURVE('',#7399,#7398,#4276,.T.);
#9371=EDGE_CURVE('',#7395,#7399,#4277,.T.);
#9372=EDGE_CURVE('',#7397,#7400,#4278,.T.);
#9373=EDGE_CURVE('',#7400,#7401,#4279,.T.);
#9374=EDGE_CURVE('',#7398,#7401,#4280,.T.);
#9375=EDGE_CURVE('',#7396,#7402,#4281,.T.);
#9376=EDGE_CURVE('',#7402,#7400,#4282,.T.);
#9377=EDGE_CURVE('',#7395,#7403,#4283,.T.);
#9378=EDGE_CURVE('',#7403,#7404,#4284,.T.);
#9379=EDGE_CURVE('',#7404,#7394,#4285,.T.);
#9380=EDGE_CURVE('',#7405,#7403,#4286,.T.);
#9381=EDGE_CURVE('',#7399,#7405,#4287,.T.);
#9382=EDGE_CURVE('',#7404,#7402,#4288,.T.);
#9383=EDGE_CURVE('',#7401,#7405,#4289,.T.);
#9384=EDGE_CURVE('',#7402,#7406,#4290,.T.);
#9385=EDGE_CURVE('',#7406,#7407,#4291,.T.);
#9386=EDGE_CURVE('',#7400,#7407,#4292,.T.);
#9387=EDGE_CURVE('',#7404,#7408,#4293,.T.);
#9388=EDGE_CURVE('',#7408,#7406,#4294,.T.);
#9389=EDGE_CURVE('',#7403,#7409,#4295,.T.);
#9390=EDGE_CURVE('',#7409,#7408,#4296,.T.);
#9391=EDGE_CURVE('',#7370,#7410,#6079,.T.);
#9392=EDGE_CURVE('',#7411,#7410,#1071,.F.);
#9393=EDGE_CURVE('',#7412,#7411,#1072,.F.);
#9394=EDGE_CURVE('',#7412,#7373,#6080,.T.);
#9395=EDGE_CURVE('',#7367,#7412,#6081,.T.);
#9396=EDGE_CURVE('',#7388,#7381,#6082,.T.);
#9397=EDGE_CURVE('',#7387,#7380,#6083,.T.);
#9398=EDGE_CURVE('',#7410,#7366,#6084,.T.);
#9399=EDGE_CURVE('',#7410,#7412,#1073,.F.);
#9400=EDGE_CURVE('',#7405,#7413,#4297,.T.);
#9401=EDGE_CURVE('',#7413,#7409,#4298,.T.);
#9402=EDGE_CURVE('',#7401,#7414,#4299,.T.);
#9403=EDGE_CURVE('',#7414,#7413,#4300,.T.);
#9404=EDGE_CURVE('',#7407,#7414,#4301,.T.);
#9405=EDGE_CURVE('',#7415,#7415,#1074,.T.);
#9406=EDGE_CURVE('',#7415,#7411,#4302,.T.);
#12806=ORIENTED_EDGE('',*,*,#9310,.F.);
#12807=ORIENTED_EDGE('',*,*,#9311,.T.);
#12808=ORIENTED_EDGE('',*,*,#9312,.T.);
#12809=ORIENTED_EDGE('',*,*,#9313,.T.);
#12810=ORIENTED_EDGE('',*,*,#9314,.F.);
#12811=ORIENTED_EDGE('',*,*,#9315,.T.);
#12812=ORIENTED_EDGE('',*,*,#9310,.T.);
#12813=ORIENTED_EDGE('',*,*,#9316,.T.);
#12814=ORIENTED_EDGE('',*,*,#9317,.F.);
#12815=ORIENTED_EDGE('',*,*,#9318,.T.);
#12816=ORIENTED_EDGE('',*,*,#9314,.T.);
#12817=ORIENTED_EDGE('',*,*,#9319,.T.);
#12818=ORIENTED_EDGE('',*,*,#9320,.F.);
#12819=ORIENTED_EDGE('',*,*,#9321,.T.);
#12820=ORIENTED_EDGE('',*,*,#9317,.T.);
#12821=ORIENTED_EDGE('',*,*,#9322,.T.);
#12822=ORIENTED_EDGE('',*,*,#9323,.F.);
#12823=ORIENTED_EDGE('',*,*,#9324,.T.);
#12824=ORIENTED_EDGE('',*,*,#9320,.T.);
#12825=ORIENTED_EDGE('',*,*,#9325,.T.);
#12826=ORIENTED_EDGE('',*,*,#9326,.F.);
#12827=ORIENTED_EDGE('',*,*,#9327,.T.);
#12828=ORIENTED_EDGE('',*,*,#9323,.T.);
#12829=ORIENTED_EDGE('',*,*,#9328,.T.);
#12830=ORIENTED_EDGE('',*,*,#9329,.F.);
#12831=ORIENTED_EDGE('',*,*,#9330,.T.);
#12832=ORIENTED_EDGE('',*,*,#9331,.F.);
#12833=ORIENTED_EDGE('',*,*,#9332,.F.);
#12834=ORIENTED_EDGE('',*,*,#9333,.T.);
#12835=ORIENTED_EDGE('',*,*,#9329,.T.);
#12836=ORIENTED_EDGE('',*,*,#9334,.F.);
#12837=ORIENTED_EDGE('',*,*,#9335,.F.);
#12838=ORIENTED_EDGE('',*,*,#9336,.F.);
#12839=ORIENTED_EDGE('',*,*,#9337,.T.);
#12840=ORIENTED_EDGE('',*,*,#9332,.T.);
#12841=ORIENTED_EDGE('',*,*,#9338,.F.);
#12842=ORIENTED_EDGE('',*,*,#9339,.F.);
#12843=ORIENTED_EDGE('',*,*,#9340,.T.);
#12844=ORIENTED_EDGE('',*,*,#9336,.T.);
#12845=ORIENTED_EDGE('',*,*,#9341,.F.);
#12846=ORIENTED_EDGE('',*,*,#9342,.F.);
#12847=ORIENTED_EDGE('',*,*,#9343,.T.);
#12848=ORIENTED_EDGE('',*,*,#9339,.T.);
#12849=ORIENTED_EDGE('',*,*,#9344,.F.);
#12850=ORIENTED_EDGE('',*,*,#9345,.F.);
#12851=ORIENTED_EDGE('',*,*,#9346,.T.);
#12852=ORIENTED_EDGE('',*,*,#9342,.T.);
#12853=ORIENTED_EDGE('',*,*,#9347,.F.);
#12854=ORIENTED_EDGE('',*,*,#9348,.T.);
#12855=ORIENTED_EDGE('',*,*,#9349,.T.);
#12856=ORIENTED_EDGE('',*,*,#9350,.T.);
#12857=ORIENTED_EDGE('',*,*,#9351,.T.);
#12858=ORIENTED_EDGE('',*,*,#9349,.F.);
#12859=ORIENTED_EDGE('',*,*,#9350,.F.);
#12860=ORIENTED_EDGE('',*,*,#9351,.F.);
#12861=ORIENTED_EDGE('',*,*,#9352,.T.);
#12862=ORIENTED_EDGE('',*,*,#9353,.F.);
#12863=ORIENTED_EDGE('',*,*,#9354,.F.);
#12864=ORIENTED_EDGE('',*,*,#9352,.F.);
#12865=ORIENTED_EDGE('',*,*,#9348,.F.);
#12866=ORIENTED_EDGE('',*,*,#9355,.T.);
#12867=ORIENTED_EDGE('',*,*,#9356,.T.);
#12868=ORIENTED_EDGE('',*,*,#9357,.T.);
#12869=ORIENTED_EDGE('',*,*,#9312,.F.);
#12870=ORIENTED_EDGE('',*,*,#9353,.T.);
#12871=ORIENTED_EDGE('',*,*,#9354,.T.);
#12872=ORIENTED_EDGE('',*,*,#9358,.T.);
#12873=ORIENTED_EDGE('',*,*,#9359,.T.);
#12874=ORIENTED_EDGE('',*,*,#9360,.T.);
#12875=ORIENTED_EDGE('',*,*,#9358,.F.);
#12876=ORIENTED_EDGE('',*,*,#9359,.F.);
#12877=ORIENTED_EDGE('',*,*,#9360,.F.);
#12878=ORIENTED_EDGE('',*,*,#9361,.T.);
#12879=ORIENTED_EDGE('',*,*,#9362,.F.);
#12880=ORIENTED_EDGE('',*,*,#9363,.F.);
#12881=ORIENTED_EDGE('',*,*,#9361,.F.);
#12882=ORIENTED_EDGE('',*,*,#9362,.T.);
#12883=ORIENTED_EDGE('',*,*,#9363,.T.);
#12884=ORIENTED_EDGE('',*,*,#9364,.T.);
#12885=ORIENTED_EDGE('',*,*,#9365,.T.);
#12886=ORIENTED_EDGE('',*,*,#9364,.F.);
#12887=ORIENTED_EDGE('',*,*,#9365,.F.);
#12888=ORIENTED_EDGE('',*,*,#9366,.F.);
#12889=ORIENTED_EDGE('',*,*,#9367,.F.);
#12890=ORIENTED_EDGE('',*,*,#9368,.F.);
#12891=ORIENTED_EDGE('',*,*,#9369,.F.);
#12892=ORIENTED_EDGE('',*,*,#9370,.F.);
#12893=ORIENTED_EDGE('',*,*,#9371,.F.);
#12894=ORIENTED_EDGE('',*,*,#9369,.T.);
#12895=ORIENTED_EDGE('',*,*,#9372,.T.);
#12896=ORIENTED_EDGE('',*,*,#9373,.T.);
#12897=ORIENTED_EDGE('',*,*,#9374,.F.);
#12898=ORIENTED_EDGE('',*,*,#9368,.T.);
#12899=ORIENTED_EDGE('',*,*,#9375,.T.);
#12900=ORIENTED_EDGE('',*,*,#9376,.T.);
#12901=ORIENTED_EDGE('',*,*,#9372,.F.);
#12902=ORIENTED_EDGE('',*,*,#9366,.T.);
#12903=ORIENTED_EDGE('',*,*,#9377,.T.);
#12904=ORIENTED_EDGE('',*,*,#9378,.T.);
#12905=ORIENTED_EDGE('',*,*,#9379,.T.);
#12906=ORIENTED_EDGE('',*,*,#9380,.T.);
#12907=ORIENTED_EDGE('',*,*,#9377,.F.);
#12908=ORIENTED_EDGE('',*,*,#9371,.T.);
#12909=ORIENTED_EDGE('',*,*,#9381,.T.);
#12910=ORIENTED_EDGE('',*,*,#9367,.T.);
#12911=ORIENTED_EDGE('',*,*,#9379,.F.);
#12912=ORIENTED_EDGE('',*,*,#9382,.T.);
#12913=ORIENTED_EDGE('',*,*,#9375,.F.);
#12914=ORIENTED_EDGE('',*,*,#9383,.T.);
#12915=ORIENTED_EDGE('',*,*,#9381,.F.);
#12916=ORIENTED_EDGE('',*,*,#9370,.T.);
#12917=ORIENTED_EDGE('',*,*,#9374,.T.);
#12918=ORIENTED_EDGE('',*,*,#9376,.F.);
#12919=ORIENTED_EDGE('',*,*,#9384,.T.);
#12920=ORIENTED_EDGE('',*,*,#9385,.T.);
#12921=ORIENTED_EDGE('',*,*,#9386,.F.);
#12922=ORIENTED_EDGE('',*,*,#9382,.F.);
#12923=ORIENTED_EDGE('',*,*,#9387,.T.);
#12924=ORIENTED_EDGE('',*,*,#9388,.T.);
#12925=ORIENTED_EDGE('',*,*,#9384,.F.);
#12926=ORIENTED_EDGE('',*,*,#9378,.F.);
#12927=ORIENTED_EDGE('',*,*,#9389,.T.);
#12928=ORIENTED_EDGE('',*,*,#9390,.T.);
#12929=ORIENTED_EDGE('',*,*,#9387,.F.);
#12930=ORIENTED_EDGE('',*,*,#9334,.T.);
#12931=ORIENTED_EDGE('',*,*,#9331,.T.);
#12932=ORIENTED_EDGE('',*,*,#9391,.T.);
#12933=ORIENTED_EDGE('',*,*,#9392,.F.);
#12934=ORIENTED_EDGE('',*,*,#9393,.F.);
#12935=ORIENTED_EDGE('',*,*,#9394,.T.);
#12936=ORIENTED_EDGE('',*,*,#9394,.F.);
#12937=ORIENTED_EDGE('',*,*,#9395,.F.);
#12938=ORIENTED_EDGE('',*,*,#9328,.F.);
#12939=ORIENTED_EDGE('',*,*,#9325,.F.);
#12940=ORIENTED_EDGE('',*,*,#9322,.F.);
#12941=ORIENTED_EDGE('',*,*,#9319,.F.);
#12942=ORIENTED_EDGE('',*,*,#9316,.F.);
#12943=ORIENTED_EDGE('',*,*,#9313,.F.);
#12944=ORIENTED_EDGE('',*,*,#9357,.F.);
#12945=ORIENTED_EDGE('',*,*,#9396,.T.);
#12946=ORIENTED_EDGE('',*,*,#9347,.T.);
#12947=ORIENTED_EDGE('',*,*,#9344,.T.);
#12948=ORIENTED_EDGE('',*,*,#9341,.T.);
#12949=ORIENTED_EDGE('',*,*,#9338,.T.);
#12950=ORIENTED_EDGE('',*,*,#9335,.T.);
#12951=ORIENTED_EDGE('',*,*,#9345,.T.);
#12952=ORIENTED_EDGE('',*,*,#9396,.F.);
#12953=ORIENTED_EDGE('',*,*,#9356,.F.);
#12954=ORIENTED_EDGE('',*,*,#9397,.T.);
#12955=ORIENTED_EDGE('',*,*,#9391,.F.);
#12956=ORIENTED_EDGE('',*,*,#9330,.F.);
#12957=ORIENTED_EDGE('',*,*,#9333,.F.);
#12958=ORIENTED_EDGE('',*,*,#9337,.F.);
#12959=ORIENTED_EDGE('',*,*,#9340,.F.);
#12960=ORIENTED_EDGE('',*,*,#9343,.F.);
#12961=ORIENTED_EDGE('',*,*,#9346,.F.);
#12962=ORIENTED_EDGE('',*,*,#9397,.F.);
#12963=ORIENTED_EDGE('',*,*,#9355,.F.);
#12964=ORIENTED_EDGE('',*,*,#9311,.F.);
#12965=ORIENTED_EDGE('',*,*,#9315,.F.);
#12966=ORIENTED_EDGE('',*,*,#9318,.F.);
#12967=ORIENTED_EDGE('',*,*,#9321,.F.);
#12968=ORIENTED_EDGE('',*,*,#9324,.F.);
#12969=ORIENTED_EDGE('',*,*,#9327,.F.);
#12970=ORIENTED_EDGE('',*,*,#9398,.F.);
#12971=ORIENTED_EDGE('',*,*,#9326,.T.);
#12972=ORIENTED_EDGE('',*,*,#9395,.T.);
#12973=ORIENTED_EDGE('',*,*,#9399,.F.);
#12974=ORIENTED_EDGE('',*,*,#9398,.T.);
#12975=ORIENTED_EDGE('',*,*,#9380,.F.);
#12976=ORIENTED_EDGE('',*,*,#9400,.T.);
#12977=ORIENTED_EDGE('',*,*,#9401,.T.);
#12978=ORIENTED_EDGE('',*,*,#9389,.F.);
#12979=ORIENTED_EDGE('',*,*,#9383,.F.);
#12980=ORIENTED_EDGE('',*,*,#9402,.T.);
#12981=ORIENTED_EDGE('',*,*,#9403,.T.);
#12982=ORIENTED_EDGE('',*,*,#9400,.F.);
#12983=ORIENTED_EDGE('',*,*,#9373,.F.);
#12984=ORIENTED_EDGE('',*,*,#9386,.T.);
#12985=ORIENTED_EDGE('',*,*,#9404,.T.);
#12986=ORIENTED_EDGE('',*,*,#9402,.F.);
#12987=ORIENTED_EDGE('',*,*,#9388,.F.);
#12988=ORIENTED_EDGE('',*,*,#9390,.F.);
#12989=ORIENTED_EDGE('',*,*,#9401,.F.);
#12990=ORIENTED_EDGE('',*,*,#9403,.F.);
#12991=ORIENTED_EDGE('',*,*,#9404,.F.);
#12992=ORIENTED_EDGE('',*,*,#9385,.F.);
#12993=ORIENTED_EDGE('',*,*,#9405,.F.);
#12994=ORIENTED_EDGE('',*,*,#9406,.T.);
#12995=ORIENTED_EDGE('',*,*,#9392,.T.);
#12996=ORIENTED_EDGE('',*,*,#9399,.T.);
#12997=ORIENTED_EDGE('',*,*,#9393,.T.);
#12998=ORIENTED_EDGE('',*,*,#9406,.F.);
#12999=ORIENTED_EDGE('',*,*,#9405,.T.);
#15827=PLANE('',#18033);
#15828=PLANE('',#18043);
#15829=PLANE('',#18044);
#15830=PLANE('',#18045);
#15831=PLANE('',#18046);
#15832=PLANE('',#18047);
#15833=PLANE('',#18048);
#15834=PLANE('',#18049);
#15835=PLANE('',#18050);
#15836=PLANE('',#18051);
#15837=PLANE('',#18052);
#15838=PLANE('',#18053);
#15839=PLANE('',#18059);
#15840=PLANE('',#18060);
#15841=PLANE('',#18061);
#15842=PLANE('',#18062);
#15843=PLANE('',#18065);
#16396=ADVANCED_FACE('',(#2225),#1425,.T.);
#16397=ADVANCED_FACE('',(#2226),#1426,.T.);
#16398=ADVANCED_FACE('',(#2227),#1427,.T.);
#16399=ADVANCED_FACE('',(#2228),#1428,.T.);
#16400=ADVANCED_FACE('',(#2229),#1429,.T.);
#16401=ADVANCED_FACE('',(#2230),#1430,.T.);
#16402=ADVANCED_FACE('',(#2231),#1431,.T.);
#16403=ADVANCED_FACE('',(#2232),#1432,.T.);
#16404=ADVANCED_FACE('',(#2233),#1433,.T.);
#16405=ADVANCED_FACE('',(#2234),#1434,.T.);
#16406=ADVANCED_FACE('',(#2235),#1435,.T.);
#16407=ADVANCED_FACE('',(#2236),#1436,.T.);
#16408=ADVANCED_FACE('',(#2237),#609,.T.);
#16409=ADVANCED_FACE('',(#2238),#1437,.T.);
#16410=ADVANCED_FACE('',(#2239,#534),#15827,.T.);
#16411=ADVANCED_FACE('',(#2240),#610,.T.);
#16412=ADVANCED_FACE('',(#2241),#611,.T.);
#16413=ADVANCED_FACE('',(#2242),#612,.T.);
#16414=ADVANCED_FACE('',(#2243,#535),#15828,.T.);
#16415=ADVANCED_FACE('',(#2244),#15829,.T.);
#16416=ADVANCED_FACE('',(#2245),#15830,.T.);
#16417=ADVANCED_FACE('',(#2246),#15831,.T.);
#16418=ADVANCED_FACE('',(#2247),#15832,.T.);
#16419=ADVANCED_FACE('',(#2248),#15833,.T.);
#16420=ADVANCED_FACE('',(#2249),#15834,.T.);
#16421=ADVANCED_FACE('',(#2250),#15835,.F.);
#16422=ADVANCED_FACE('',(#2251),#15836,.F.);
#16423=ADVANCED_FACE('',(#2252),#15837,.F.);
#16424=ADVANCED_FACE('',(#2253),#15838,.F.);
#16425=ADVANCED_FACE('',(#2254),#353,.F.);
#16426=ADVANCED_FACE('',(#2255),#1438,.T.);
#16427=ADVANCED_FACE('',(#2256),#354,.F.);
#16428=ADVANCED_FACE('',(#2257),#1439,.T.);
#16429=ADVANCED_FACE('',(#2258),#15839,.F.);
#16430=ADVANCED_FACE('',(#2259),#15840,.F.);
#16431=ADVANCED_FACE('',(#2260),#15841,.F.);
#16432=ADVANCED_FACE('',(#2261),#15842,.F.);
#16433=ADVANCED_FACE('',(#2262),#613,.T.);
#16434=ADVANCED_FACE('',(#2263),#15843,.T.);
#16959=CLOSED_SHELL('',(#16396,#16397,#16398,#16399,#16400,#16401,#16402,
#16403,#16404,#16405,#16406,#16407,#16408,#16409,#16410,#16411,#16412,#16413,
#16414,#16415,#16416,#16417,#16418,#16419,#16420,#16421,#16422,#16423,#16424,
#16425,#16426,#16427,#16428,#16429,#16430,#16431,#16432,#16433,#16434));
#18010=AXIS2_PLACEMENT_3D('',#34065,#20783,#20784);
#18011=AXIS2_PLACEMENT_3D('',#34066,#20785,#20786);
#18012=AXIS2_PLACEMENT_3D('',#34088,#20788,#20789);
#18013=AXIS2_PLACEMENT_3D('',#34099,#20790,#20791);
#18014=AXIS2_PLACEMENT_3D('',#34183,#20793,#20794);
#18015=AXIS2_PLACEMENT_3D('',#34273,#20796,#20797);
#18016=AXIS2_PLACEMENT_3D('',#34357,#20799,#20800);
#18017=AXIS2_PLACEMENT_3D('',#34447,#20802,#20803);
#18018=AXIS2_PLACEMENT_3D('',#34537,#20805,#20806);
#18019=AXIS2_PLACEMENT_3D('',#34546,#20808,#20809);
#18020=AXIS2_PLACEMENT_3D('',#34547,#20810,#20811);
#18021=AXIS2_PLACEMENT_3D('',#34569,#20813,#20814);
#18022=AXIS2_PLACEMENT_3D('',#34584,#20815,#20816);
#18023=AXIS2_PLACEMENT_3D('',#34622,#20818,#20819);
#18024=AXIS2_PLACEMENT_3D('',#34659,#20821,#20822);
#18025=AXIS2_PLACEMENT_3D('',#34696,#20824,#20825);
#18026=AXIS2_PLACEMENT_3D('',#34733,#20827,#20828);
#18027=AXIS2_PLACEMENT_3D('',#34735,#20829,#20830);
#18028=AXIS2_PLACEMENT_3D('',#34739,#20832,#20833);
#18029=AXIS2_PLACEMENT_3D('',#34740,#20834,#20835);
#18030=AXIS2_PLACEMENT_3D('',#34741,#20836,#20837);
#18031=AXIS2_PLACEMENT_3D('',#34745,#20839,#20840);
#18032=AXIS2_PLACEMENT_3D('',#34746,#20841,#20842);
#18033=AXIS2_PLACEMENT_3D('',#34747,#20843,#20844);
#18034=AXIS2_PLACEMENT_3D('',#34883,#20845,#20846);
#18035=AXIS2_PLACEMENT_3D('',#35017,#20847,#20848);
#18036=AXIS2_PLACEMENT_3D('',#35021,#20850,#20851);
#18037=AXIS2_PLACEMENT_3D('',#35022,#20852,#20853);
#18038=AXIS2_PLACEMENT_3D('',#35023,#20854,#20855);
#18039=AXIS2_PLACEMENT_3D('',#35027,#20857,#20858);
#18040=AXIS2_PLACEMENT_3D('',#35028,#20859,#20860);
#18041=AXIS2_PLACEMENT_3D('',#35029,#20861,#20862);
#18042=AXIS2_PLACEMENT_3D('',#35032,#20864,#20865);
#18043=AXIS2_PLACEMENT_3D('',#35033,#20866,#20867);
#18044=AXIS2_PLACEMENT_3D('',#35046,#20874,#20875);
#18045=AXIS2_PLACEMENT_3D('',#35052,#20879,#20880);
#18046=AXIS2_PLACEMENT_3D('',#35056,#20883,#20884);
#18047=AXIS2_PLACEMENT_3D('',#35062,#20888,#20889);
#18048=AXIS2_PLACEMENT_3D('',#35066,#20892,#20893);
#18049=AXIS2_PLACEMENT_3D('',#35068,#20895,#20896);
#18050=AXIS2_PLACEMENT_3D('',#35070,#20898,#20899);
#18051=AXIS2_PLACEMENT_3D('',#35076,#20903,#20904);
#18052=AXIS2_PLACEMENT_3D('',#35080,#20907,#20908);
#18053=AXIS2_PLACEMENT_3D('',#35084,#20911,#20912);
#18054=AXIS2_PLACEMENT_3D('',#35220,#20913,#20914);
#18055=AXIS2_PLACEMENT_3D('',#35222,#20915,#20916);
#18056=AXIS2_PLACEMENT_3D('',#35708,#20917,#20918);
#18057=AXIS2_PLACEMENT_3D('',#36053,#20919,#20920);
#18058=AXIS2_PLACEMENT_3D('',#36054,#20921,#20922);
#18059=AXIS2_PLACEMENT_3D('',#36055,#20923,#20924);
#18060=AXIS2_PLACEMENT_3D('',#36059,#20927,#20928);
#18061=AXIS2_PLACEMENT_3D('',#36063,#20931,#20932);
#18062=AXIS2_PLACEMENT_3D('',#36065,#20934,#20935);
#18063=AXIS2_PLACEMENT_3D('',#36066,#20936,#20937);
#18064=AXIS2_PLACEMENT_3D('',#36068,#20938,#20939);
#18065=AXIS2_PLACEMENT_3D('',#36070,#20941,#20942);
#20783=DIRECTION('axis',(0.,0.,1.));
#20784=DIRECTION('refdir',(1.,0.,0.));
#20785=DIRECTION('center_axis',(1.,0.,0.));
#20786=DIRECTION('ref_axis',(0.,1.,0.));
#20787=DIRECTION('',(-1.,0.,0.));
#20788=DIRECTION('center_axis',(-1.,0.,0.));
#20789=DIRECTION('ref_axis',(0.,1.,0.));
#20790=DIRECTION('center_axis',(1.,0.,0.));
#20791=DIRECTION('ref_axis',(0.,1.,0.));
#20792=DIRECTION('',(-1.,0.,0.));
#20793=DIRECTION('center_axis',(1.,0.,0.));
#20794=DIRECTION('ref_axis',(0.,1.,0.));
#20795=DIRECTION('',(-1.,0.,0.));
#20796=DIRECTION('center_axis',(1.,0.,0.));
#20797=DIRECTION('ref_axis',(0.,1.,0.));
#20798=DIRECTION('',(-1.,0.,0.));
#20799=DIRECTION('center_axis',(1.,0.,0.));
#20800=DIRECTION('ref_axis',(0.,1.,0.));
#20801=DIRECTION('',(-1.,0.,0.));
#20802=DIRECTION('center_axis',(1.,0.,0.));
#20803=DIRECTION('ref_axis',(0.,1.,0.));
#20804=DIRECTION('',(-1.,0.,0.));
#20805=DIRECTION('center_axis',(1.,0.,0.));
#20806=DIRECTION('ref_axis',(0.,-0.979063397301506,-0.203555555228623));
#20807=DIRECTION('',(1.,0.,0.));
#20808=DIRECTION('center_axis',(1.,0.,0.));
#20809=DIRECTION('ref_axis',(0.,1.,4.09245417118841E-15));
#20810=DIRECTION('center_axis',(1.,0.,0.));
#20811=DIRECTION('ref_axis',(0.,1.,4.09245417118841E-15));
#20812=DIRECTION('',(1.,0.,0.));
#20813=DIRECTION('center_axis',(1.,0.,0.));
#20814=DIRECTION('ref_axis',(0.,1.,4.09245417118841E-15));
#20815=DIRECTION('center_axis',(1.,0.,0.));
#20816=DIRECTION('ref_axis',(0.,1.,4.09245417118841E-15));
#20817=DIRECTION('',(1.,0.,0.));
#20818=DIRECTION('center_axis',(1.,0.,0.));
#20819=DIRECTION('ref_axis',(0.,1.,4.09245417118841E-15));
#20820=DIRECTION('',(1.,0.,0.));
#20821=DIRECTION('center_axis',(1.,0.,0.));
#20822=DIRECTION('ref_axis',(0.,1.,4.09245417118841E-15));
#20823=DIRECTION('',(1.,0.,0.));
#20824=DIRECTION('center_axis',(1.,0.,0.));
#20825=DIRECTION('ref_axis',(0.,1.,4.09245417118841E-15));
#20826=DIRECTION('',(1.,0.,0.));
#20827=DIRECTION('center_axis',(-1.,0.,0.));
#20828=DIRECTION('ref_axis',(0.,-1.,0.));
#20829=DIRECTION('center_axis',(-1.,0.,0.));
#20830=DIRECTION('ref_axis',(0.,-1.,0.));
#20831=DIRECTION('',(-0.707106781186552,0.707106781186543,8.65956056235488E-17));
#20832=DIRECTION('center_axis',(1.,0.,0.));
#20833=DIRECTION('ref_axis',(0.,-1.,0.));
#20834=DIRECTION('center_axis',(1.,0.,0.));
#20835=DIRECTION('ref_axis',(0.,-1.,0.));
#20836=DIRECTION('center_axis',(1.,0.,0.));
#20837=DIRECTION('ref_axis',(0.,1.,0.));
#20838=DIRECTION('',(-1.,0.,0.));
#20839=DIRECTION('center_axis',(-1.,0.,0.));
#20840=DIRECTION('ref_axis',(0.,-1.,0.));
#20841=DIRECTION('center_axis',(-1.,0.,0.));
#20842=DIRECTION('ref_axis',(0.,-1.,0.));
#20843=DIRECTION('center_axis',(1.,0.,0.));
#20844=DIRECTION('ref_axis',(0.,0.,-1.));
#20845=DIRECTION('center_axis',(-1.,0.,0.));
#20846=DIRECTION('ref_axis',(0.,1.,4.09245417118841E-15));
#20847=DIRECTION('center_axis',(1.,0.,1.12244711165176E-15));
#20848=DIRECTION('ref_axis',(0.,-1.,-3.02741268154642E-17));
#20849=DIRECTION('',(-0.923879532511291,-0.38268343236508,-1.09545652359634E-15));
#20850=DIRECTION('center_axis',(1.,0.,0.));
#20851=DIRECTION('ref_axis',(0.,-1.,-6.12323399573677E-17));
#20852=DIRECTION('center_axis',(1.,0.,0.));
#20853=DIRECTION('ref_axis',(0.,-1.,-6.12323399573677E-17));
#20854=DIRECTION('center_axis',(1.,0.,0.));
#20855=DIRECTION('ref_axis',(0.,1.,0.));
#20856=DIRECTION('',(-0.707106781186546,0.707106781186549,8.65956056235495E-17));
#20857=DIRECTION('center_axis',(-1.,0.,0.));
#20858=DIRECTION('ref_axis',(0.,-1.,-6.12323399573677E-17));
#20859=DIRECTION('center_axis',(-1.,0.,0.));
#20860=DIRECTION('ref_axis',(0.,-1.,-6.12323399573677E-17));
#20861=DIRECTION('center_axis',(1.,0.,-2.65910050866385E-15));
#20862=DIRECTION('ref_axis',(0.,-1.,-3.14915276069828E-17));
#20863=DIRECTION('',(-0.382683432365087,-0.923879532511288,8.75356720626856E-16));
#20864=DIRECTION('center_axis',(1.,0.,0.));
#20865=DIRECTION('ref_axis',(0.,-1.,0.));
#20866=DIRECTION('center_axis',(-1.,0.,0.));
#20867=DIRECTION('ref_axis',(0.,0.,1.));
#20868=DIRECTION('',(0.,-0.866025403784439,-0.5));
#20869=DIRECTION('',(0.,-3.84592537276713E-16,-1.));
#20870=DIRECTION('',(0.,0.866025403784439,-0.5));
#20871=DIRECTION('',(0.,0.866025403784439,0.5));
#20872=DIRECTION('',(0.,-1.92296268638356E-16,1.));
#20873=DIRECTION('',(0.,-0.866025403784439,0.5));
#20874=DIRECTION('center_axis',(-0.707106781186546,0.353553390593275,-0.612372435695796));
#20875=DIRECTION('ref_axis',(-0.654653670707979,0.,0.755928946018453));
#20876=DIRECTION('',(0.654653670707981,6.27736560906509E-15,-0.755928946018451));
#20877=DIRECTION('',(0.,-0.866025403784439,-0.5));
#20878=DIRECTION('',(0.65465367070798,0.654653670707973,-0.377964473009229));
#20879=DIRECTION('center_axis',(-0.707106781186543,-0.353553390593276,-0.612372435695799));
#20880=DIRECTION('ref_axis',(-0.654653670707982,0.,0.75592894601845));
#20881=DIRECTION('',(0.654653670707982,-0.654653670707975,-0.377964473009223));
#20882=DIRECTION('',(0.,-0.866025403784439,0.5));
#20883=DIRECTION('center_axis',(-0.707106781186543,-0.353553390593276,0.612372435695799));
#20884=DIRECTION('ref_axis',(0.654653670707983,0.,0.75592894601845));
#20885=DIRECTION('',(0.654653670707981,3.69906210244107E-15,0.755928946018451));
#20886=DIRECTION('',(0.,0.866025403784439,0.5));
#20887=DIRECTION('',(-0.654653670707982,0.654653670707974,-0.377964473009224));
#20888=DIRECTION('center_axis',(-0.707106781186545,0.353553390593275,0.612372435695797));
#20889=DIRECTION('ref_axis',(0.65465367070798,0.,0.755928946018452));
#20890=DIRECTION('',(0.,0.866025403784439,-0.5));
#20891=DIRECTION('',(0.654653670707981,0.654653670707973,0.377964473009228));
#20892=DIRECTION('center_axis',(-0.707106781186543,-0.707106781186552,2.71947991102105E-16));
#20893=DIRECTION('ref_axis',(3.84592537276717E-16,0.,1.));
#20894=DIRECTION('',(0.,3.84592537276713E-16,1.));
#20895=DIRECTION('center_axis',(-0.707106781186544,0.707106781186551,1.35973995551053E-16));
#20896=DIRECTION('ref_axis',(1.92296268638359E-16,0.,1.));
#20897=DIRECTION('',(0.,1.92296268638356E-16,-1.));
#20898=DIRECTION('center_axis',(0.,0.5,0.866025403784439));
#20899=DIRECTION('ref_axis',(0.,-0.866025403784439,0.5));
#20900=DIRECTION('',(1.,0.,0.));
#20901=DIRECTION('',(0.,-0.866025403784439,0.5));
#20902=DIRECTION('',(1.,0.,0.));
#20903=DIRECTION('center_axis',(0.,1.,-3.84592537276713E-16));
#20904=DIRECTION('ref_axis',(0.,3.84592537276713E-16,1.));
#20905=DIRECTION('',(1.,0.,0.));
#20906=DIRECTION('',(0.,3.84592537276713E-16,1.));
#20907=DIRECTION('center_axis',(0.,0.5,-0.866025403784439));
#20908=DIRECTION('ref_axis',(0.,0.866025403784439,0.5));
#20909=DIRECTION('',(1.,0.,0.));
#20910=DIRECTION('',(0.,0.866025403784439,0.5));
#20911=DIRECTION('center_axis',(1.,0.,0.));
#20912=DIRECTION('ref_axis',(0.,0.,-1.));
#20913=DIRECTION('center_axis',(-1.,0.,0.));
#20914=DIRECTION('ref_axis',(0.,1.,0.));
#20915=DIRECTION('center_axis',(-1.,0.,0.));
#20916=DIRECTION('ref_axis',(0.,1.,0.));
#20917=DIRECTION('center_axis',(1.,0.,0.));
#20918=DIRECTION('ref_axis',(0.,0.888972258373966,0.457961050572524));
#20919=DIRECTION('center_axis',(1.,0.,0.));
#20920=DIRECTION('ref_axis',(0.,0.117347197905867,-0.993090950086467));
#20921=DIRECTION('center_axis',(-1.,0.,0.));
#20922=DIRECTION('ref_axis',(0.,1.,0.));
#20923=DIRECTION('center_axis',(0.,-0.5,-0.866025403784439));
#20924=DIRECTION('ref_axis',(0.,0.866025403784439,-0.5));
#20925=DIRECTION('',(1.,0.,0.));
#20926=DIRECTION('',(0.,0.866025403784439,-0.5));
#20927=DIRECTION('center_axis',(0.,-1.,-1.92296268638356E-16));
#20928=DIRECTION('ref_axis',(0.,1.92296268638356E-16,-1.));
#20929=DIRECTION('',(1.,0.,0.));
#20930=DIRECTION('',(0.,1.92296268638356E-16,-1.));
#20931=DIRECTION('center_axis',(0.,-0.5,0.866025403784439));
#20932=DIRECTION('ref_axis',(0.,-0.866025403784439,-0.5));
#20933=DIRECTION('',(0.,-0.866025403784439,-0.5));
#20934=DIRECTION('center_axis',(1.,0.,0.));
#20935=DIRECTION('ref_axis',(0.,0.,-1.));
#20936=DIRECTION('center_axis',(-1.,0.,0.));
#20937=DIRECTION('ref_axis',(0.,1.,0.));
#20938=DIRECTION('center_axis',(1.,0.,0.));
#20939=DIRECTION('ref_axis',(0.,0.,-1.));
#20940=DIRECTION('',(-0.707106781186552,-0.707106781186543,-8.65956056235488E-17));
#20941=DIRECTION('center_axis',(1.,0.,0.));
#20942=DIRECTION('ref_axis',(0.,0.,-1.));
#34065=CARTESIAN_POINT('',(0.,0.,0.));
#34066=CARTESIAN_POINT('Origin',(-85.75,0.,0.));
#34067=CARTESIAN_POINT('',(-89.5188431528481,-11.9252862155783,0.000296729823191094));
#34068=CARTESIAN_POINT('',(-89.7311568471519,-11.9248987907529,0.000229507259365661));
#34069=CARTESIAN_POINT('',(-85.75,-11.925,-1.46039130798322E-15));
#34070=CARTESIAN_POINT('',(-90.,5.1296446118907,10.7653319110792));
#34071=CARTESIAN_POINT('Ctrl Pts',(-89.5188431528481,-11.9252862155783,
0.000296729823191094));
#34072=CARTESIAN_POINT('Ctrl Pts',(-89.5262732725778,-11.9256675610804,
0.37140882978507));
#34073=CARTESIAN_POINT('Ctrl Pts',(-89.5337033923074,-11.9086887659417,
0.742486110439695));
#34074=CARTESIAN_POINT('Ctrl Pts',(-89.5411335120371,-11.874094865106,1.11191379148113));
#34075=CARTESIAN_POINT('Ctrl Pts',(-89.5809184802334,-11.6888599974842,
3.09003380513459));
#34076=CARTESIAN_POINT('Ctrl Pts',(-89.6207034484296,-10.9985782879942,
5.02085775997829));
#34077=CARTESIAN_POINT('Ctrl Pts',(-89.6604884166259,-9.88773523873562,
6.66807012563771));
#34078=CARTESIAN_POINT('Ctrl Pts',(-89.7002733848221,-8.77689218947705,
8.31528249129713));
#34079=CARTESIAN_POINT('Ctrl Pts',(-89.7400583530184,-7.24548780044994,
9.67888326777227));
#34080=CARTESIAN_POINT('Ctrl Pts',(-89.7798433212147,-5.48096071686973,
10.5919600041883));
#34081=CARTESIAN_POINT('Ctrl Pts',(-89.8196282894109,-3.71643363328953,
11.5050367406042));
#34082=CARTESIAN_POINT('Ctrl Pts',(-89.8594132576072,-1.71878385515623,
11.967589436961));
#34083=CARTESIAN_POINT('Ctrl Pts',(-89.8991982258034,0.267492608476263,
11.9230350042462));
#34084=CARTESIAN_POINT('Ctrl Pts',(-89.9327988172023,1.94501220659287,11.8854063380305));
#34085=CARTESIAN_POINT('Ctrl Pts',(-89.9663994086011,3.61441952603868,11.4860718254948));
#34086=CARTESIAN_POINT('Ctrl Pts',(-90.,5.13009691060871,10.7656670051304));
#34087=CARTESIAN_POINT('',(-90.,-5.1296446118933,10.765331911078));
#34088=CARTESIAN_POINT('Origin',(-90.,0.,0.));
#34089=CARTESIAN_POINT('Ctrl Pts',(-90.,-5.12964461189318,10.765331911078));
#34090=CARTESIAN_POINT('Ctrl Pts',(-89.9602150318037,-6.92369670303529,
9.91047209636926));
#34091=CARTESIAN_POINT('Ctrl Pts',(-89.9204300636075,-8.49893930959995,
8.59874522586898));
#34092=CARTESIAN_POINT('Ctrl Pts',(-89.8806450954112,-9.66327664795995,
6.98920240711812));
#34093=CARTESIAN_POINT('Ctrl Pts',(-89.840860127215,-10.8276139863199,5.37965958836726));
#34094=CARTESIAN_POINT('Ctrl Pts',(-89.8010751590187,-11.5810460564753,
3.47230082136582));
#34095=CARTESIAN_POINT('Ctrl Pts',(-89.7612901908224,-11.831183536793,1.50127032371404));
#34096=CARTESIAN_POINT('Ctrl Pts',(-89.7512457429322,-11.8943353501623,
1.00364737662614));
#34097=CARTESIAN_POINT('Ctrl Pts',(-89.741201295042,-11.9254070149145,0.501965974265288));
#34098=CARTESIAN_POINT('Ctrl Pts',(-89.7311568471519,-11.9248987907529,
0.000229507259365661));
#34099=CARTESIAN_POINT('Origin',(-85.75,0.,0.));
#34100=CARTESIAN_POINT('',(-88.0188431528482,-11.9249138545732,-0.000313305576115086));
#34101=CARTESIAN_POINT('',(-88.2311568471518,-11.9253287759226,-0.000290940587986354));
#34102=CARTESIAN_POINT('',(-85.75,-11.925,-1.46039130798322E-15));
#34103=CARTESIAN_POINT('Ctrl Pts',(-88.0188431528482,-11.9249138545732,
-0.000313305576115086));
#34104=CARTESIAN_POINT('Ctrl Pts',(-88.0488536542227,-11.9233842134251,
1.49875571795511));
#34105=CARTESIAN_POINT('Ctrl Pts',(-88.0788641555972,-11.6398512903311,
2.99838693882232));
#34106=CARTESIAN_POINT('Ctrl Pts',(-88.1088746569718,-11.0879741656425,
4.39173220896684));
#34107=CARTESIAN_POINT('Ctrl Pts',(-88.148659625168,-10.3563498058901,6.23889219364382));
#34108=CARTESIAN_POINT('Ctrl Pts',(-88.1884445933643,-9.15311464423924,
7.89925625669109));
#34109=CARTESIAN_POINT('Ctrl Pts',(-88.2282295615605,-7.62553833621686,
9.16960457008304));
#34110=CARTESIAN_POINT('Ctrl Pts',(-88.2680145297567,-6.09796202819448,
10.439952883475));
#34111=CARTESIAN_POINT('Ctrl Pts',(-88.307799497953,-4.24604457380059,11.3202854472116));
#34112=CARTESIAN_POINT('Ctrl Pts',(-88.3475844661493,-2.29645093028959,
11.7028541830264));
#34113=CARTESIAN_POINT('Ctrl Pts',(-88.3873694343455,-0.346857286778581,
12.0854229188411));
#34114=CARTESIAN_POINT('Ctrl Pts',(-88.4271544025418,1.70041254584955,11.9702278267339));
#34115=CARTESIAN_POINT('Ctrl Pts',(-88.4669393707381,3.59478350797716,11.3713681849374));
#34116=CARTESIAN_POINT('Ctrl Pts',(-88.5067243389343,5.48915447010478,10.7725085431409));
#34117=CARTESIAN_POINT('Ctrl Pts',(-88.5465093071305,7.23062656173189,9.68998435165513));
#34118=CARTESIAN_POINT('Ctrl Pts',(-88.5862942753268,8.60605275571365,8.25629086835593));
#34119=CARTESIAN_POINT('Ctrl Pts',(-88.626079243523,9.9814789496954,6.82259738505672));
#34120=CARTESIAN_POINT('Ctrl Pts',(-88.6658642117193,10.9908592460318,5.03773460994408));
#34121=CARTESIAN_POINT('Ctrl Pts',(-88.7056491799156,11.5106508088721,3.12016038042581));
#34122=CARTESIAN_POINT('Ctrl Pts',(-88.7454341481119,12.0304423717123,1.20258615090756));
#34123=CARTESIAN_POINT('Ctrl Pts',(-88.7852191163081,12.0606452010564,-0.847699533016319));
#34124=CARTESIAN_POINT('Ctrl Pts',(-88.8250040845044,11.5975626213517,-2.77975252944092));
#34125=CARTESIAN_POINT('Ctrl Pts',(-88.8647890527006,11.134480041647,-4.71180552586556));
#34126=CARTESIAN_POINT('Ctrl Pts',(-88.9045740208969,10.1781120528935,-6.52562583479092));
#34127=CARTESIAN_POINT('Ctrl Pts',(-88.9443589890932,8.84551308397863,-7.99921130042105));
#34128=CARTESIAN_POINT('Ctrl Pts',(-88.9841439572895,7.51291411506383,-9.47279676605115));
#34129=CARTESIAN_POINT('Ctrl Pts',(-89.0239289254857,5.80408416598773,-10.606147388386));
#34130=CARTESIAN_POINT('Ctrl Pts',(-89.0637138936819,3.92817500056627,-11.2605471970953));
#34131=CARTESIAN_POINT('Ctrl Pts',(-89.1034988618782,2.05226583514479,-11.9149470058045));
#34132=CARTESIAN_POINT('Ctrl Pts',(-89.1432838300745,0.00927745337794966,
-12.0903960008881));
#34133=CARTESIAN_POINT('Ctrl Pts',(-89.1830687982707,-1.95073903883306,
-11.7654197631003));
#34134=CARTESIAN_POINT('Ctrl Pts',(-89.222853766467,-3.91075553104407,-11.4404435253125));
#34135=CARTESIAN_POINT('Ctrl Pts',(-89.2626387346633,-5.78780013369925,
-10.6150420546534));
#34136=CARTESIAN_POINT('Ctrl Pts',(-89.3024237028595,-7.35213260967356,
-9.39024094984122));
#34137=CARTESIAN_POINT('Ctrl Pts',(-89.3422086710558,-8.91646508564786,
-8.16543984502907));
#34138=CARTESIAN_POINT('Ctrl Pts',(-89.381993639252,-10.1680854349413,-6.54123910606394));
#34139=CARTESIAN_POINT('Ctrl Pts',(-89.4217786074483,-10.9538015967113,
-4.71643070034976));
#34140=CARTESIAN_POINT('Ctrl Pts',(-89.4541334559149,-11.5927797963778,
-3.23241796578538));
#34141=CARTESIAN_POINT('Ctrl Pts',(-89.4864883043815,-11.9236256264652,
-1.61573049386844));
#34142=CARTESIAN_POINT('Ctrl Pts',(-89.5188431528481,-11.9252862155783,
0.000296729823191094));
#34143=CARTESIAN_POINT('Ctrl Pts',(-89.7311568471519,-11.9248987907529,
0.000229507259365661));
#34144=CARTESIAN_POINT('Ctrl Pts',(-89.7014163268458,-11.9233939941566,
-1.48535772943447));
#34145=CARTESIAN_POINT('Ctrl Pts',(-89.6716758065397,-11.6450321505873,
-2.9714277111775));
#34146=CARTESIAN_POINT('Ctrl Pts',(-89.6419352862337,-11.1027988892476,
-4.35406132175854));
#34147=CARTESIAN_POINT('Ctrl Pts',(-89.6021503180374,-10.3774338709044,
-6.20366024127725));
#34148=CARTESIAN_POINT('Ctrl Pts',(-89.5623653498411,-9.17986094373797,
-7.86815585201252));
#34149=CARTESIAN_POINT('Ctrl Pts',(-89.5225803816448,-7.65660908602565,
-9.14369467174216));
#34150=CARTESIAN_POINT('Ctrl Pts',(-89.4827954134486,-6.13335722831333,
-10.4192334914718));
#34151=CARTESIAN_POINT('Ctrl Pts',(-89.4430104452524,-4.28442644005515,
-11.3058155201958));
#34152=CARTESIAN_POINT('Ctrl Pts',(-89.4032254770561,-2.3361391875209,-11.6949890221749));
#34153=CARTESIAN_POINT('Ctrl Pts',(-89.3634405088599,-0.387851934986667,
-12.0841625241539));
#34154=CARTESIAN_POINT('Ctrl Pts',(-89.3236555406636,1.65979178182363,-11.975927499388));
#34155=CARTESIAN_POINT('Ctrl Pts',(-89.2838705724673,3.55618223645511,-11.3835018375421));
#34156=CARTESIAN_POINT('Ctrl Pts',(-89.244085604271,5.45257269108659,-10.7910761756962));
#34157=CARTESIAN_POINT('Ctrl Pts',(-89.2043006360747,7.19770988353926,-9.71445987677028));
#34158=CARTESIAN_POINT('Ctrl Pts',(-89.1645156678785,8.57799285603494,-8.28543931996323));
#34159=CARTESIAN_POINT('Ctrl Pts',(-89.1247306996822,9.95827582853063,-6.85641876315616));
#34160=CARTESIAN_POINT('Ctrl Pts',(-89.084945731486,10.9737045810693,-5.07499394846794));
#34161=CARTESIAN_POINT('Ctrl Pts',(-89.0451607632897,11.4999985475621,-3.15919506363862));
#34162=CARTESIAN_POINT('Ctrl Pts',(-89.0053757950935,12.0262925140549,-1.2433961788093));
#34163=CARTESIAN_POINT('Ctrl Pts',(-88.9655908268973,12.0634516945017,0.806776776161122));
#34164=CARTESIAN_POINT('Ctrl Pts',(-88.925805858701,11.6069267617573,2.74039011995642));
#34165=CARTESIAN_POINT('Ctrl Pts',(-88.8860208905047,11.150401829013,4.6740034637517));
#34166=CARTESIAN_POINT('Ctrl Pts',(-88.8462359223084,10.2001927830774,6.49105719637186));
#34167=CARTESIAN_POINT('Ctrl Pts',(-88.8064509541121,8.87260081037856,7.96915508324411));
#34168=CARTESIAN_POINT('Ctrl Pts',(-88.7666659859158,7.5450088376797,9.44725297011637));
#34169=CARTESIAN_POINT('Ctrl Pts',(-88.7268810177196,5.84003393821749,10.5863950112407));
#34170=CARTESIAN_POINT('Ctrl Pts',(-88.6870960495234,3.96635578564482,11.2471554480454));
#34171=CARTESIAN_POINT('Ctrl Pts',(-88.6473110813271,2.09267763307216,11.9079158848501));
#34172=CARTESIAN_POINT('Ctrl Pts',(-88.6075261131309,0.0502962273890387,
12.0902947173352));
#34173=CARTESIAN_POINT('Ctrl Pts',(-88.5677411449346,-1.91081155032196,
11.7719701033081));
#34174=CARTESIAN_POINT('Ctrl Pts',(-88.5279561767384,-3.87191932803296,
11.453645489281));
#34175=CARTESIAN_POINT('Ctrl Pts',(-88.4881712085421,-5.75175347777183,
10.6346174287416));
#34176=CARTESIAN_POINT('Ctrl Pts',(-88.4483862403458,-7.32023225262676,
9.41513047179962));
#34177=CARTESIAN_POINT('Ctrl Pts',(-88.4086012721495,-8.88871102748168,
8.19564351485764));
#34178=CARTESIAN_POINT('Ctrl Pts',(-88.3688163039533,-10.1458344274527,
6.57569766151304));
#34179=CARTESIAN_POINT('Ctrl Pts',(-88.3290313357571,-10.9377371277736,
4.75356584986406));
#34180=CARTESIAN_POINT('Ctrl Pts',(-88.296406506222,-11.5871203440395,3.2593648377581));
#34181=CARTESIAN_POINT('Ctrl Pts',(-88.2637816766869,-11.9236670000931,
1.62920435573443));
#34182=CARTESIAN_POINT('Ctrl Pts',(-88.2311568471518,-11.9253287759226,
-0.000290940587986354));
#34183=CARTESIAN_POINT('Origin',(-85.75,0.,0.));
#34184=CARTESIAN_POINT('',(-86.5188431528481,-11.9244727711418,0.000275034636322557));
#34185=CARTESIAN_POINT('',(-86.7311568471519,-11.9241833131278,0.00019535608514432));
#34186=CARTESIAN_POINT('',(-85.75,-11.925,-1.46039130798322E-15));
#34187=CARTESIAN_POINT('Ctrl Pts',(-86.5188431528481,-11.9244727711418,
0.000275034636322557));
#34188=CARTESIAN_POINT('Ctrl Pts',(-86.5316490676713,-11.925012519502,0.640017395537692));
#34189=CARTESIAN_POINT('Ctrl Pts',(-86.5444549824944,-11.8744209897277,
1.27967524169772));
#34190=CARTESIAN_POINT('Ctrl Pts',(-86.5572608973175,-11.771953842827,1.9109122468146));
#34191=CARTESIAN_POINT('Ctrl Pts',(-86.5970458655138,-11.4536124953399,
3.87201729239096));
#34192=CARTESIAN_POINT('Ctrl Pts',(-86.6368308337101,-10.6345682683525,
5.75184447388234));
#34193=CARTESIAN_POINT('Ctrl Pts',(-86.6766158019064,-9.41506786773371,
7.32031283065446));
#34194=CARTESIAN_POINT('Ctrl Pts',(-86.7164007701026,-8.1955674671149,8.88878118742658));
#34195=CARTESIAN_POINT('Ctrl Pts',(-86.7561857382989,-6.57561089286461,
10.1458907194795));
#34196=CARTESIAN_POINT('Ctrl Pts',(-86.7959707064951,-4.75347231000134,
10.9377778314759));
#34197=CARTESIAN_POINT('Ctrl Pts',(-86.8357556746914,-2.93133372713806,
11.7296649434723));
#34198=CARTESIAN_POINT('Ctrl Pts',(-86.8755406428876,-0.907013135661791,
12.0563296354123));
#34199=CARTESIAN_POINT('Ctrl Pts',(-86.9153256110839,1.07172327033036,11.8777898669959));
#34200=CARTESIAN_POINT('Ctrl Pts',(-86.9551105792802,3.0504596763225,11.6992500985794));
#34201=CARTESIAN_POINT('Ctrl Pts',(-86.9948955474764,4.98361189683049,11.0155058698065));
#34202=CARTESIAN_POINT('Ctrl Pts',(-87.0346805156727,6.63457226689149,9.9102438783345));
#34203=CARTESIAN_POINT('Ctrl Pts',(-87.0744654838689,8.28553263695249,8.80498188686248));
#34204=CARTESIAN_POINT('Ctrl Pts',(-87.1142504520652,9.6543011565665,7.27820213269135));
#34205=CARTESIAN_POINT('Ctrl Pts',(-87.1540354202615,10.573347757555,5.51677442809552));
#34206=CARTESIAN_POINT('Ctrl Pts',(-87.1938203884578,11.4923943585434,3.75534672349969));
#34207=CARTESIAN_POINT('Ctrl Pts',(-87.233605356654,11.9617190409063,1.75927106847916));
#34208=CARTESIAN_POINT('Ctrl Pts',(-87.2733903248502,11.9238789317937,-0.227143374542267));
#34209=CARTESIAN_POINT('Ctrl Pts',(-87.3131752930465,11.8860388226812,-2.21355781756369));
#34210=CARTESIAN_POINT('Ctrl Pts',(-87.3529602612428,11.3410339220931,-4.19031104858601));
#34211=CARTESIAN_POINT('Ctrl Pts',(-87.392745229439,10.3555699635724,-5.91545886827222));
#34212=CARTESIAN_POINT('Ctrl Pts',(-87.4325301976353,9.37010600505178,-7.64060668795844));
#34213=CARTESIAN_POINT('Ctrl Pts',(-87.4723151658315,7.94418298859856,-9.11414909630856));
#34214=CARTESIAN_POINT('Ctrl Pts',(-87.5121001340278,6.25232639222003,-10.1557322521756));
#34215=CARTESIAN_POINT('Ctrl Pts',(-87.551885102224,4.56046979584153,-11.1973154080427));
#34216=CARTESIAN_POINT('Ctrl Pts',(-87.5916700704203,2.60267961953774,-11.8069393114268));
#34217=CARTESIAN_POINT('Ctrl Pts',(-87.6314550386166,0.618579084479763,
-11.9099892027141));
#34218=CARTESIAN_POINT('Ctrl Pts',(-87.6712400068129,-1.36552145057824,
-12.0130390940015));
#34219=CARTESIAN_POINT('Ctrl Pts',(-87.7110249750091,-3.37593234439042,
-11.6095149731922));
#34220=CARTESIAN_POINT('Ctrl Pts',(-87.7508099432054,-5.16658987668869,
-10.748806070401));
#34221=CARTESIAN_POINT('Ctrl Pts',(-87.7905949114016,-6.95724740898696,
-9.88809716760979));
#34222=CARTESIAN_POINT('Ctrl Pts',(-87.8303798795979,-8.52815157977131,
-8.57020348283671));
#34223=CARTESIAN_POINT('Ctrl Pts',(-87.8701648477942,-9.68703198025464,
-6.95642827216015));
#34224=CARTESIAN_POINT('Ctrl Pts',(-87.9099498159904,-10.845912380738,-5.34265306148359));
#34225=CARTESIAN_POINT('Ctrl Pts',(-87.9497347841867,-11.5927690109203,
-3.43299632490356));
#34226=CARTESIAN_POINT('Ctrl Pts',(-87.9895197523829,-11.8361905470845,
-1.46119000346019));
#34227=CARTESIAN_POINT('Ctrl Pts',(-87.9992942192047,-11.8959949364508,
-0.976751876658961));
#34228=CARTESIAN_POINT('Ctrl Pts',(-88.0090686860264,-11.9254120610665,
-0.488562410485842));
#34229=CARTESIAN_POINT('Ctrl Pts',(-88.0188431528482,-11.9249138545732,
-0.000313305576115086));
#34230=CARTESIAN_POINT('Ctrl Pts',(-88.2311568471518,-11.9253287759226,
-0.000290940587986354));
#34231=CARTESIAN_POINT('Ctrl Pts',(-88.2239967084906,-11.9256934841995,
-0.357914641177949));
#34232=CARTESIAN_POINT('Ctrl Pts',(-88.2168365698294,-11.9099279125869,
-0.715506302006868));
#34233=CARTESIAN_POINT('Ctrl Pts',(-88.2096764311682,-11.8777989864306,
-1.07162165229349));
#34234=CARTESIAN_POINT('Ctrl Pts',(-88.169891462972,-11.6992761440956,-3.05035957284871));
#34235=CARTESIAN_POINT('Ctrl Pts',(-88.1301064947758,-11.0155484587548,
-4.98351764400581));
#34236=CARTESIAN_POINT('Ctrl Pts',(-88.0903215265795,-9.91030059580027,
-6.63448746494451));
#34237=CARTESIAN_POINT('Ctrl Pts',(-88.0505365583832,-8.80505273284578,
-8.28545728588321));
#34238=CARTESIAN_POINT('Ctrl Pts',(-88.010751590187,-7.27828469227764,-9.65423885660352));
#34239=CARTESIAN_POINT('Ctrl Pts',(-87.9709666219907,-5.51686485626861,
-10.5733005210593));
#34240=CARTESIAN_POINT('Ctrl Pts',(-87.9311816537944,-3.75544502025959,
-11.492362185515));
#34241=CARTESIAN_POINT('Ctrl Pts',(-87.8913966855982,-1.75937338880969,
-11.9617039437062));
#34242=CARTESIAN_POINT('Ctrl Pts',(-87.8516117174019,0.227041369848316,
-11.9238808282072));
#34243=CARTESIAN_POINT('Ctrl Pts',(-87.8118267492057,2.21345612850632,-11.8860577127083));
#34244=CARTESIAN_POINT('Ctrl Pts',(-87.7720417810094,4.19021401437242,-11.3410697235191));
#34245=CARTESIAN_POINT('Ctrl Pts',(-87.7322568128131,5.91537025754448,-10.3556205265248));
#34246=CARTESIAN_POINT('Ctrl Pts',(-87.6924718446169,7.64052650071656,-9.37017132953037));
#34247=CARTESIAN_POINT('Ctrl Pts',(-87.6526868764206,9.11408110119458,-7.94426092473072));
#34248=CARTESIAN_POINT('Ctrl Pts',(-87.6129019082243,10.1556787259928,-6.25241324546769));
#34249=CARTESIAN_POINT('Ctrl Pts',(-87.5731169400281,11.1972763507911,-4.56056556620466));
#34250=CARTESIAN_POINT('Ctrl Pts',(-87.5333319718319,11.8069169999095,-2.60278061247826));
#34251=CARTESIAN_POINT('Ctrl Pts',(-87.4935470036356,11.9099838639235,-0.618680966760705));
#34252=CARTESIAN_POINT('Ctrl Pts',(-87.4537620354393,12.0130507279375,1.36541867895684));
#34253=CARTESIAN_POINT('Ctrl Pts',(-87.413977067243,11.6095438068471,3.37583301666555));
#34254=CARTESIAN_POINT('Ctrl Pts',(-87.3741920990468,10.7488502257642,5.16649790484009));
#34255=CARTESIAN_POINT('Ctrl Pts',(-87.3344071308505,9.88815664468133,6.95716279301464));
#34256=CARTESIAN_POINT('Ctrl Pts',(-87.2946221626543,8.57027640360599,8.52807823165505));
#34257=CARTESIAN_POINT('Ctrl Pts',(-87.2548371944581,6.95651111301019,9.68697243270591));
#34258=CARTESIAN_POINT('Ctrl Pts',(-87.2150522262618,5.34274582241438,10.8458666337568));
#34259=CARTESIAN_POINT('Ctrl Pts',(-87.1752672580655,3.4330954822981,11.5927395972181));
#34260=CARTESIAN_POINT('Ctrl Pts',(-87.1354822898692,1.46129125108685,11.8361780003709));
#34261=CARTESIAN_POINT('Ctrl Pts',(-87.0956973216729,-0.510512980124398,
12.0796164035238));
#34262=CARTESIAN_POINT('Ctrl Pts',(-87.0559123534767,-2.54447110243062,
11.8196202463681));
#34263=CARTESIAN_POINT('Ctrl Pts',(-87.0161273852804,-4.3916373386571,11.0880116911415));
#34264=CARTESIAN_POINT('Ctrl Pts',(-86.9763424170842,-6.23880357488359,
10.3564031359149));
#34265=CARTESIAN_POINT('Ctrl Pts',(-86.936557448888,-7.89917792503034,9.15318218261725));
#34266=CARTESIAN_POINT('Ctrl Pts',(-86.8967724806917,-9.16953930086925,
7.6256167479702));
#34267=CARTESIAN_POINT('Ctrl Pts',(-86.8569875124955,-10.4399006767081,
6.09805131332317));
#34268=CARTESIAN_POINT('Ctrl Pts',(-86.8172025442992,-11.3202490782392,
4.24614139732673));
#34269=CARTESIAN_POINT('Ctrl Pts',(-86.7774175761029,-11.7028344910425,
2.29655103413447));
#34270=CARTESIAN_POINT('Ctrl Pts',(-86.7619973331192,-11.851120647722,1.54090993444184));
#34271=CARTESIAN_POINT('Ctrl Pts',(-86.7465770901356,-11.9246299821493,
0.770594715534088));
#34272=CARTESIAN_POINT('Ctrl Pts',(-86.7311568471519,-11.9241833131278,
0.00019535608514432));
#34273=CARTESIAN_POINT('Origin',(-85.75,0.,0.));
#34274=CARTESIAN_POINT('',(-85.0188431528481,-11.9257267375167,-0.000211608777844763));
#34275=CARTESIAN_POINT('',(-85.2311568471519,-11.9259825692636,-9.38362929313221E-5));
#34276=CARTESIAN_POINT('',(-85.75,-11.925,-1.46039130798322E-15));
#34277=CARTESIAN_POINT('Ctrl Pts',(-85.0188431528481,-11.9257267375167,
-0.000211608777844763));
#34278=CARTESIAN_POINT('Ctrl Pts',(-85.0542294493162,-11.9242705478464,
1.7670388487699));
#34279=CARTESIAN_POINT('Ctrl Pts',(-85.0896157457842,-11.5263826191068,
3.53492306196897));
#34280=CARTESIAN_POINT('Ctrl Pts',(-85.1250020422522,-10.7662288870872,
5.13018503014497));
#34281=CARTESIAN_POINT('Ctrl Pts',(-85.1647870104484,-9.91158471487207,
6.92374505205773));
#34282=CARTESIAN_POINT('Ctrl Pts',(-85.2045719786447,-8.5990147066321,8.49910013949158));
#34283=CARTESIAN_POINT('Ctrl Pts',(-85.244356946841,-6.98917052831226,9.66343511484645));
#34284=CARTESIAN_POINT('Ctrl Pts',(-85.2841419150372,-5.37932634999243,
10.8277700902013));
#34285=CARTESIAN_POINT('Ctrl Pts',(-85.3239268832335,-3.47220800159274,
11.5810849534772));
#34286=CARTESIAN_POINT('Ctrl Pts',(-85.3637118514297,-1.50123673904742,
11.83117792724));
#34287=CARTESIAN_POINT('Ctrl Pts',(-85.403496819626,0.469734523497902,12.0812709010027));
#34288=CARTESIAN_POINT('Ctrl Pts',(-85.4432817878222,2.50455870018884,11.8281419852523));
#34289=CARTESIAN_POINT('Ctrl Pts',(-85.4830667560185,4.35418401333848,11.102772828022));
#34290=CARTESIAN_POINT('Ctrl Pts',(-85.5228517242148,6.20380932648811,10.3774036707916));
#34291=CARTESIAN_POINT('Ctrl Pts',(-85.562636692411,7.86823577609642,9.17979427208133));
#34292=CARTESIAN_POINT('Ctrl Pts',(-85.6024216606073,9.14374631827695,7.65652572383014));
#34293=CARTESIAN_POINT('Ctrl Pts',(-85.6422066288036,10.4192568604575,6.13325717557897));
#34294=CARTESIAN_POINT('Ctrl Pts',(-85.6819915969998,11.3058514952102,4.28432947778694));
#34295=CARTESIAN_POINT('Ctrl Pts',(-85.7217765651961,11.6950157020167,2.33604165678988));
#34296=CARTESIAN_POINT('Ctrl Pts',(-85.7615615333924,12.0841799088233,0.38775383579276));
#34297=CARTESIAN_POINT('Ctrl Pts',(-85.8013465015887,11.9759136876837,-1.65989410840939));
#34298=CARTESIAN_POINT('Ctrl Pts',(-85.8411314697849,11.383468254672,-3.55628083642892));
#34299=CARTESIAN_POINT('Ctrl Pts',(-85.8809164379812,10.7910228216603,-5.4526675644484));
#34300=CARTESIAN_POINT('Ctrl Pts',(-85.9207014061774,9.71439817677659,-7.19779307628529));
#34301=CARTESIAN_POINT('Ctrl Pts',(-85.9604863743736,8.28536751437418,-8.57806318724856));
#34302=CARTESIAN_POINT('Ctrl Pts',(-86.0002713425699,6.85633685197174,-9.95833329821186));
#34303=CARTESIAN_POINT('Ctrl Pts',(-86.0400563107662,5.07490017205052,-10.9737480083016));
#34304=CARTESIAN_POINT('Ctrl Pts',(-86.0798412789624,3.15909595530759,-11.500025897268));
#34305=CARTESIAN_POINT('Ctrl Pts',(-86.1196262471587,1.24329173856466,-12.0263037862345));
#34306=CARTESIAN_POINT('Ctrl Pts',(-86.1594112153549,-0.806880015000012,
-12.0634448540777));
#34307=CARTESIAN_POINT('Ctrl Pts',(-86.1991961835512,-2.74048906500605,
-11.6069032294259));
#34308=CARTESIAN_POINT('Ctrl Pts',(-86.2389811517475,-4.67409811501208,
-11.1503616047741));
#34309=CARTESIAN_POINT('Ctrl Pts',(-86.2787661199437,-6.49114446145946,
-10.2001372876273));
#34310=CARTESIAN_POINT('Ctrl Pts',(-86.31855108814,-7.96923118774666,-8.8725327369879));
#34311=CARTESIAN_POINT('Ctrl Pts',(-86.3583360563363,-9.44731791403387,
-7.54492818634847));
#34312=CARTESIAN_POINT('Ctrl Pts',(-86.3981210245325,-10.5864450201609,
-5.83994340221645));
#34313=CARTESIAN_POINT('Ctrl Pts',(-86.4379059927288,-11.247189339231,-3.96625955531976));
#34314=CARTESIAN_POINT('Ctrl Pts',(-86.4648850461019,-11.6952544517187,
-2.69567373354868));
#34315=CARTESIAN_POINT('Ctrl Pts',(-86.491864099475,-11.923335648178,-1.34751179185571));
#34316=CARTESIAN_POINT('Ctrl Pts',(-86.5188431528481,-11.9244727711418,
0.000275034636322557));
#34317=CARTESIAN_POINT('Ctrl Pts',(-86.7311568471519,-11.9241833131278,
0.00019535608514432));
#34318=CARTESIAN_POINT('Ctrl Pts',(-86.7067921219393,-11.923477554601,-1.21707266730429));
#34319=CARTESIAN_POINT('Ctrl Pts',(-86.6824273967267,-11.7381367941709,
-2.43455075192281));
#34320=CARTESIAN_POINT('Ctrl Pts',(-86.6580626715141,-11.3713988928199,
-3.59468621683454));
#34321=CARTESIAN_POINT('Ctrl Pts',(-86.6182777033178,-10.7725554577184,
-5.48906229422317));
#34322=CARTESIAN_POINT('Ctrl Pts',(-86.5784927351216,-9.69004616343957,
-7.23054363861233));
#34323=CARTESIAN_POINT('Ctrl Pts',(-86.5387077669254,-8.25636445447486,
-8.60598209224268));
#34324=CARTESIAN_POINT('Ctrl Pts',(-86.4989227987291,-6.82268274551014,
-9.98142054587304));
#34325=CARTESIAN_POINT('Ctrl Pts',(-86.4591378305328,-5.0378286218595,-10.9908161087446));
#34326=CARTESIAN_POINT('Ctrl Pts',(-86.4193528623365,-3.12025884135912,
-11.5106240725707));
#34327=CARTESIAN_POINT('Ctrl Pts',(-86.3795678941403,-1.20268906085873,
-12.0304320363968));
#34328=CARTESIAN_POINT('Ctrl Pts',(-86.3397829259441,0.847596376491398,
-12.0606524011774));
#34329=CARTESIAN_POINT('Ctrl Pts',(-86.2999979577478,2.77965331601329,-11.5975863531985));
#34330=CARTESIAN_POINT('Ctrl Pts',(-86.2602129895515,4.71171025553519,-11.1345203052197));
#34331=CARTESIAN_POINT('Ctrl Pts',(-86.2204280213552,6.52553869722884,-10.1781678444814));
#34332=CARTESIAN_POINT('Ctrl Pts',(-86.180643053159,7.99913557911104,-8.84558148253248));
#34333=CARTESIAN_POINT('Ctrl Pts',(-86.1408580849627,9.47273246099324,-7.51299512058353));
#34334=CARTESIAN_POINT('Ctrl Pts',(-86.1010731167665,10.606097783064,-5.80417485742391));
#34335=CARTESIAN_POINT('Ctrl Pts',(-86.0612881485702,11.2605135904926,-3.92827130624306));
#34336=CARTESIAN_POINT('Ctrl Pts',(-86.021503180374,11.9149293979212,-2.05236775506224));
#34337=CARTESIAN_POINT('Ctrl Pts',(-85.9817182121776,12.0903956907077,-0.00938091586017931));
#34338=CARTESIAN_POINT('Ctrl Pts',(-85.9419332439814,11.7654363174268,1.95063836671386));
#34339=CARTESIAN_POINT('Ctrl Pts',(-85.9021482757851,11.4404769441458,3.91065764928794));
#34340=CARTESIAN_POINT('Ctrl Pts',(-85.8623633075889,10.6150919047974,5.78770937523399));
#34341=CARTESIAN_POINT('Ctrl Pts',(-85.8225783393926,9.3903039873357,7.35205228507991));
#34342=CARTESIAN_POINT('Ctrl Pts',(-85.7827933711964,8.165516069874,8.91639519492582));
#34343=CARTESIAN_POINT('Ctrl Pts',(-85.7430084030001,6.54132527429904,10.1680292886716));
#34344=CARTESIAN_POINT('Ctrl Pts',(-85.7032234348038,4.71652401205079,10.9537611358323));
#34345=CARTESIAN_POINT('Ctrl Pts',(-85.6634384666076,2.89172274980254,11.739492982993));
#34346=CARTESIAN_POINT('Ctrl Pts',(-85.6236534984113,0.866311020881004,
12.0593225835686));
#34347=CARTESIAN_POINT('Ctrl Pts',(-85.5838685302151,-1.1118114311319,11.8741044764953));
#34348=CARTESIAN_POINT('Ctrl Pts',(-85.5440835620188,-3.0899338831448,11.688886369422));
#34349=CARTESIAN_POINT('Ctrl Pts',(-85.5042985938226,-5.02076705824908,
10.9986205546999));
#34350=CARTESIAN_POINT('Ctrl Pts',(-85.4645136256263,-6.66798713044286,
9.88779193780744));
#34351=CARTESIAN_POINT('Ctrl Pts',(-85.4247286574301,-8.31520720263664,
8.77696332091496));
#34352=CARTESIAN_POINT('Ctrl Pts',(-85.3849436892338,-9.67881417191992,
7.24557190185211));
#34353=CARTESIAN_POINT('Ctrl Pts',(-85.3451587210375,-10.5919097167293,
5.48105193642395));
#34354=CARTESIAN_POINT('Ctrl Pts',(-85.3071580964089,-11.4640532076362,
3.79567014787885));
#34355=CARTESIAN_POINT('Ctrl Pts',(-85.2691574717804,-11.9251896698631,
1.8976023630708));
#34356=CARTESIAN_POINT('Ctrl Pts',(-85.2311568471519,-11.9259825692636,
-9.38362929313221E-5));
#34357=CARTESIAN_POINT('Origin',(-85.75,0.,0.));
#34358=CARTESIAN_POINT('',(-83.5188431528481,-11.9240088006309,7.96196756353007E-5));
#34359=CARTESIAN_POINT('',(-83.7311568471519,-11.9239866250219,-4.23754525262851E-5));
#34360=CARTESIAN_POINT('',(-85.75,-11.925,-1.46039130798322E-15));
#34361=CARTESIAN_POINT('Ctrl Pts',(-83.5188431528481,-11.9240088006309,
7.96196756353007E-5));
#34362=CARTESIAN_POINT('Ctrl Pts',(-83.5370248627648,-11.9242195872713,
0.908480640254555));
#34363=CARTESIAN_POINT('Ctrl Pts',(-83.5552065726814,-11.8217585988444,
1.81683486812291));
#34364=CARTESIAN_POINT('Ctrl Pts',(-83.573388282598,-11.6161109140083,2.70119420587685));
#34365=CARTESIAN_POINT('Ctrl Pts',(-83.6131732507943,-11.166115471426,4.63633717581385));
#34366=CARTESIAN_POINT('Ctrl Pts',(-83.6529582189906,-10.2220456992873,
6.45658879193667));
#34367=CARTESIAN_POINT('Ctrl Pts',(-83.6927431871868,-8.89945077497426,
7.93915982913878));
#34368=CARTESIAN_POINT('Ctrl Pts',(-83.7325281553831,-7.57685585066127,
9.42173086634086));
#34369=CARTESIAN_POINT('Ctrl Pts',(-83.7723131235793,-5.87573577417402,
10.5666213246222));
#34370=CARTESIAN_POINT('Ctrl Pts',(-83.8120980917756,-4.00429869523271,
11.2337026332634));
#34371=CARTESIAN_POINT('Ctrl Pts',(-83.8518830599718,-2.13286161629138,
11.9007839419046));
#34372=CARTESIAN_POINT('Ctrl Pts',(-83.8916680281681,-0.0911075348959658,
12.0900561009056));
#34373=CARTESIAN_POINT('Ctrl Pts',(-83.9314529963644,1.87106358683858,11.7783531933421));
#34374=CARTESIAN_POINT('Ctrl Pts',(-83.9712379645607,3.83323470857312,11.4666502857785));
#34375=CARTESIAN_POINT('Ctrl Pts',(-84.0110229327569,5.7158228706468,10.6539723116505));
#34376=CARTESIAN_POINT('Ctrl Pts',(-84.0508079009531,7.28840918318163,9.4397867809977));
#34377=CARTESIAN_POINT('Ctrl Pts',(-84.0905928691494,8.86099549571648,8.22560125034485));
#34378=CARTESIAN_POINT('Ctrl Pts',(-84.1303778373456,10.1235799587125,6.60990816316717));
#34379=CARTESIAN_POINT('Ctrl Pts',(-84.1701628055419,10.9216288739539,4.79045985606893));
#34380=CARTESIAN_POINT('Ctrl Pts',(-84.2099477737382,11.7196777891953,2.97101154897075));
#34381=CARTESIAN_POINT('Ctrl Pts',(-84.2497327419345,12.0531911566822,0.94780802195201));
#34382=CARTESIAN_POINT('Ctrl Pts',(-84.2895177101307,11.8813486943064,-1.03152125369576));
#34383=CARTESIAN_POINT('Ctrl Pts',(-84.329302678327,11.7095062319307,-3.01085052934356));
#34384=CARTESIAN_POINT('Ctrl Pts',(-84.3690876465232,11.0323079396923,-4.94630555362038));
#34385=CARTESIAN_POINT('Ctrl Pts',(-84.4088726147195,9.93263932701359,-6.60099681049727));
#34386=CARTESIAN_POINT('Ctrl Pts',(-84.4486575829157,8.83297071433485,-8.25568806737415));
#34387=CARTESIAN_POINT('Ctrl Pts',(-84.488442551112,7.31083178121576,-9.62961555685108));
#34388=CARTESIAN_POINT('Ctrl Pts',(-84.5282275193082,5.55252432785638,-10.5546177799685));
#34389=CARTESIAN_POINT('Ctrl Pts',(-84.5680124875045,3.794216874497,-11.4796200030859));
#34390=CARTESIAN_POINT('Ctrl Pts',(-84.6077974557008,1.79974090089733,-11.9556969598438));
#34391=CARTESIAN_POINT('Ctrl Pts',(-84.6475824238971,-0.186790223121584,
-11.9245793345182));
#34392=CARTESIAN_POINT('Ctrl Pts',(-84.6873673920933,-2.1733213471405,-11.8934617091927));
#34393=CARTESIAN_POINT('Ctrl Pts',(-84.7271523602896,-4.15190762157867,
-11.3551495017836));
#34394=CARTESIAN_POINT('Ctrl Pts',(-84.7669373284859,-5.88038049221546,
-10.3755292953879));
#34395=CARTESIAN_POINT('Ctrl Pts',(-84.8067222966821,-7.60885336285225,
-9.3959090889922));
#34396=CARTESIAN_POINT('Ctrl Pts',(-84.8465072648784,-9.08721282968765,
-7.97498088360977));
#34397=CARTESIAN_POINT('Ctrl Pts',(-84.8862922330746,-10.1345154689654,
-6.28665881863918));
#34398=CARTESIAN_POINT('Ctrl Pts',(-84.9260772012709,-11.1818181082431,
-4.59833675366858));
#34399=CARTESIAN_POINT('Ctrl Pts',(-84.9658621694672,-11.7980639199631,
-2.64262082910982));
#34400=CARTESIAN_POINT('Ctrl Pts',(-85.0056471376634,-11.9078276577279,
-0.658880388634596));
#34401=CARTESIAN_POINT('Ctrl Pts',(-85.0100458093917,-11.9199632625049,
-0.439555769631561));
#34402=CARTESIAN_POINT('Ctrl Pts',(-85.0144444811199,-11.9259077482744,
-0.219888585467614));
#34403=CARTESIAN_POINT('Ctrl Pts',(-85.0188431528481,-11.9257267375167,
-0.000211608777844763));
#34404=CARTESIAN_POINT('Ctrl Pts',(-85.2311568471519,-11.9259825692636,
-9.38362929313221E-5));
#34405=CARTESIAN_POINT('Ctrl Pts',(-85.2293725035842,-11.9260198003607,
-0.0892013717583456));
#34406=CARTESIAN_POINT('Ctrl Pts',(-85.2275881600165,-11.9250420512741,
-0.17830808794031));
#34407=CARTESIAN_POINT('Ctrl Pts',(-85.2258038164487,-11.9230442142274,
-0.267391927138796));
#34408=CARTESIAN_POINT('Ctrl Pts',(-85.1860188482525,-11.8784990465807,
-2.25366731347994));
#34409=CARTESIAN_POINT('Ctrl Pts',(-85.1462338800562,-11.3268245909518,
-4.22856957436877));
#34410=CARTESIAN_POINT('Ctrl Pts',(-85.1064489118599,-10.3355428993453,
-5.95038105947133));
#34411=CARTESIAN_POINT('Ctrl Pts',(-85.0666639436637,-9.34426120773877,
-7.6721925445739));
#34412=CARTESIAN_POINT('Ctrl Pts',(-85.0268789754674,-7.9133722801547,-9.14091325389021));
#34413=CARTESIAN_POINT('Ctrl Pts',(-84.9870940072712,-6.21800939600349,
-10.1767794968906));
#34414=CARTESIAN_POINT('Ctrl Pts',(-84.947309039075,-4.52264651185229,-11.212645739891));
#34415=CARTESIAN_POINT('Ctrl Pts',(-84.9075240708787,-2.56280967113394,
-11.8156575165756));
#34416=CARTESIAN_POINT('Ctrl Pts',(-84.8677391026824,-0.578372595985458,
-11.9120093568354));
#34417=CARTESIAN_POINT('Ctrl Pts',(-84.8279541344861,1.40606447916304,-12.0083611970952));
#34418=CARTESIAN_POINT('Ctrl Pts',(-84.7881691662899,3.41510178874168,-11.5980531009304));
#34419=CARTESIAN_POINT('Ctrl Pts',(-84.7483841980936,5.20284373197974,-10.7313046214205));
#34420=CARTESIAN_POINT('Ctrl Pts',(-84.7085992298973,6.99058567521779,-9.86455614191062));
#34421=CARTESIAN_POINT('Ctrl Pts',(-84.6688142617011,8.55703225211528,-8.54136727905574));
#34422=CARTESIAN_POINT('Ctrl Pts',(-84.6290292935048,9.71045863991032,-6.92368939075921));
#34423=CARTESIAN_POINT('Ctrl Pts',(-84.5892443253086,10.8638850277054,-5.30601150246268));
#34424=CARTESIAN_POINT('Ctrl Pts',(-84.5494593571123,11.6042912263979,-3.39384458872447));
#34425=CARTESIAN_POINT('Ctrl Pts',(-84.509674388916,11.8410554112094,-1.4212278233248));
#34426=CARTESIAN_POINT('Ctrl Pts',(-84.4698894207198,12.0778195960208,0.551388942074894));
#34427=CARTESIAN_POINT('Ctrl Pts',(-84.4301044525235,11.8109417669511,2.58445555913603));
#34428=CARTESIAN_POINT('Ctrl Pts',(-84.3903194843273,11.0730863667161,4.42913536622702));
#34429=CARTESIAN_POINT('Ctrl Pts',(-84.350534516131,10.3352309664812,6.27381517331799));
#34430=CARTESIAN_POINT('Ctrl Pts',(-84.3107495479347,9.12639799508108,7.93010817043879));
#34431=CARTESIAN_POINT('Ctrl Pts',(-84.2709645797385,7.59454225072356,9.19529280551203));
#34432=CARTESIAN_POINT('Ctrl Pts',(-84.2311796115422,6.06268650636603,10.4604774405853));
#34433=CARTESIAN_POINT('Ctrl Pts',(-84.191394643346,4.20780798905109,11.334553713611));
#34434=CARTESIAN_POINT('Ctrl Pts',(-84.1516096751497,2.25693407413093,11.7105392857095));
#34435=CARTESIAN_POINT('Ctrl Pts',(-84.1118247069535,0.30606015921078,12.086524857808));
#34436=CARTESIAN_POINT('Ctrl Pts',(-84.0720397387572,-1.74080915331459,
11.9644197289793));
#34437=CARTESIAN_POINT('Ctrl Pts',(-84.032254770561,-3.63314782448661,11.3591689248174));
#34438=CARTESIAN_POINT('Ctrl Pts',(-83.9924698023647,-5.52548649565861,
10.7539181206555));
#34439=CARTESIAN_POINT('Ctrl Pts',(-83.9526848341684,-7.26329452547726,
9.66552164116037));
#34440=CARTESIAN_POINT('Ctrl Pts',(-83.9128998659722,-8.63387335055236,
8.22719349133102));
#34441=CARTESIAN_POINT('Ctrl Pts',(-83.8731148977759,-10.0044521756275,
6.78886534150164));
#34442=CARTESIAN_POINT('Ctrl Pts',(-83.8333299295796,-11.0078017959591,
5.00060552133803));
#34443=CARTESIAN_POINT('Ctrl Pts',(-83.7935449613834,-11.5211174948606,
3.0812876280193));
#34444=CARTESIAN_POINT('Ctrl Pts',(-83.7727489233062,-11.7894332257493,
2.07803917009065));
#34445=CARTESIAN_POINT('Ctrl Pts',(-83.751952885229,-11.9238585928665,1.03898214397406));
#34446=CARTESIAN_POINT('Ctrl Pts',(-83.7311568471519,-11.9239866250219,
-4.23754525262852E-5));
#34447=CARTESIAN_POINT('Origin',(-85.75,0.,0.));
#34448=CARTESIAN_POINT('',(-82.0188431528482,-11.9260172048445,5.30405712340781E-5));
#34449=CARTESIAN_POINT('',(-82.2311568471519,-11.9258224962353,0.000178908662697473));
#34450=CARTESIAN_POINT('',(-85.75,-11.925,-1.46039130798322E-15));
#34451=CARTESIAN_POINT('Ctrl Pts',(-82.0188431528482,-11.9260172048445,
5.30405712340781E-5));
#34452=CARTESIAN_POINT('Ctrl Pts',(-82.0198202762134,-11.9260288816802,
0.0488487122931931));
#34453=CARTESIAN_POINT('Ctrl Pts',(-82.0207973995787,-11.925735492526,0.0976442386766466));
#34454=CARTESIAN_POINT('Ctrl Pts',(-82.0217745229439,-11.9251361629207,
0.146436006056953));
#34455=CARTESIAN_POINT('Ctrl Pts',(-82.0615594911402,-11.900733605235,2.13306224232621));
#34456=CARTESIAN_POINT('Ctrl Pts',(-82.1013444593364,-11.3691346776982,
4.1134567013229));
#34457=CARTESIAN_POINT('Ctrl Pts',(-82.1411294275327,-10.3953731816262,
5.84523425748872));
#34458=CARTESIAN_POINT('Ctrl Pts',(-82.1809143957289,-9.42161168555416,
7.57701181365452));
#34459=CARTESIAN_POINT('Ctrl Pts',(-82.2206993639251,-8.00568762094685,
9.06017246698947));
#34460=CARTESIAN_POINT('Ctrl Pts',(-82.2604843321214,-6.32091762223773,
10.1131828701275));
#34461=CARTESIAN_POINT('Ctrl Pts',(-82.3002693003177,-4.63614762352858,
11.1661932732656));
#34462=CARTESIAN_POINT('Ctrl Pts',(-82.340054268514,-2.68253169071761,11.7890534262067));
#34463=CARTESIAN_POINT('Ctrl Pts',(-82.3798392367102,-0.699174929923869,
11.9055296212553));
#34464=CARTESIAN_POINT('Ctrl Pts',(-82.4196242049065,1.28418183086987,12.0220058163039));
#34465=CARTESIAN_POINT('Ctrl Pts',(-82.4594091731028,3.29727941964638,11.6320980534599));
#34466=CARTESIAN_POINT('Ctrl Pts',(-82.499194141299,5.09372180800857,10.7835284630743));
#34467=CARTESIAN_POINT('Ctrl Pts',(-82.5389791094953,6.89016419637075,9.9349588726887));
#34468=CARTESIAN_POINT('Ctrl Pts',(-82.5787640776915,8.46995138431862,8.62772745476145));
#34469=CARTESIAN_POINT('Ctrl Pts',(-82.6185490458878,9.63972739936108,7.02183271463421));
#34470=CARTESIAN_POINT('Ctrl Pts',(-82.658334014084,10.8095034144035,5.41593797450697));
#34471=CARTESIAN_POINT('Ctrl Pts',(-82.6981189822803,11.5692682565406,3.51137991217972));
#34472=CARTESIAN_POINT('Ctrl Pts',(-82.7379039504766,11.8260299004481,1.54126629538404));
#34473=CARTESIAN_POINT('Ctrl Pts',(-82.7776889186728,12.0827915443555,-0.428847321411644));
#34474=CARTESIAN_POINT('Ctrl Pts',(-82.8174738868691,11.8365499900335,-2.46451649267577));
#34475=CARTESIAN_POINT('Ctrl Pts',(-82.8572588550654,11.1174442959487,-4.31658595878279));
#34476=CARTESIAN_POINT('Ctrl Pts',(-82.8970438232616,10.398338601864,-6.1686554248898));
#34477=CARTESIAN_POINT('Ctrl Pts',(-82.9368287914578,9.20636876801659,-7.83712518583971));
#34478=CARTESIAN_POINT('Ctrl Pts',(-82.9766137596541,7.68742544683738,-9.11778334612848));
#34479=CARTESIAN_POINT('Ctrl Pts',(-83.0163987278503,6.16848212565817,-10.3984415064173));
#34480=CARTESIAN_POINT('Ctrl Pts',(-83.0561836960466,4.32256531714715,-11.2912880660449));
#34481=CARTESIAN_POINT('Ctrl Pts',(-83.0959686642429,2.37560562037672,-11.6870432880836));
#34482=CARTESIAN_POINT('Ctrl Pts',(-83.1357536324391,0.4286459236063,-12.0827985101224));
#34483=CARTESIAN_POINT('Ctrl Pts',(-83.1755386006354,-1.61935666142352,
-11.9814623945722));
#34484=CARTESIAN_POINT('Ctrl Pts',(-83.2153235688317,-3.51773743235987,
-11.395437955618));
#34485=CARTESIAN_POINT('Ctrl Pts',(-83.255108537028,-5.41611820329623,-10.8094135166638));
#34486=CARTESIAN_POINT('Ctrl Pts',(-83.2948935052242,-7.1648771601391,-9.73870075430558));
#34487=CARTESIAN_POINT('Ctrl Pts',(-83.3346784734205,-8.54997538283724,
-8.31434927639566));
#34488=CARTESIAN_POINT('Ctrl Pts',(-83.3744634416168,-9.93507360553538,
-6.88999779848573));
#34489=CARTESIAN_POINT('Ctrl Pts',(-83.414248409813,-10.9565110940888,-5.1120076050241));
#34490=CARTESIAN_POINT('Ctrl Pts',(-83.4540333780092,-11.4892692818526,
-3.19799534641771));
#34491=CARTESIAN_POINT('Ctrl Pts',(-83.4756366362888,-11.7785572529796,
-2.15868570140124));
#34492=CARTESIAN_POINT('Ctrl Pts',(-83.4972398945685,-11.9237583468368,
-1.07927001020106));
#34493=CARTESIAN_POINT('Ctrl Pts',(-83.5188431528481,-11.9240088006309,
7.96196756353007E-5));
#34494=CARTESIAN_POINT('Ctrl Pts',(-83.7311568471519,-11.9239866250219,
-4.23754525262852E-5));
#34495=CARTESIAN_POINT('Ctrl Pts',(-83.7121679170328,-11.9241035316002,
-0.948779049150204));
#34496=CARTESIAN_POINT('Ctrl Pts',(-83.6931789869137,-11.8122490199285,
-1.89748862014936));
#34497=CARTESIAN_POINT('Ctrl Pts',(-83.6741900567946,-11.588113260095,-2.8188850364372));
#34498=CARTESIAN_POINT('Ctrl Pts',(-83.6344050885983,-11.1185115489563,
-4.74936384110115));
#34499=CARTESIAN_POINT('Ctrl Pts',(-83.5946201204021,-10.1560263492076,
-6.55994548395522));
#34500=CARTESIAN_POINT('Ctrl Pts',(-83.5548351522058,-8.81846078752594,
-8.02902429411543));
#34501=CARTESIAN_POINT('Ctrl Pts',(-83.5150501840096,-7.48089522584431,
-9.49810310427565));
#34502=CARTESIAN_POINT('Ctrl Pts',(-83.4752652158133,-5.76824930222981,
-10.625679081742));
#34503=CARTESIAN_POINT('Ctrl Pts',(-83.435480247617,-3.89014187032842,-11.2737428570226));
#34504=CARTESIAN_POINT('Ctrl Pts',(-83.3956952794208,-2.01203443842704,
-11.9218066323032));
#34505=CARTESIAN_POINT('Ctrl Pts',(-83.3559103112245,0.0315345017612198,
-12.090358205398));
#34506=CARTESIAN_POINT('Ctrl Pts',(-83.3161253430283,1.99044285894123,-11.7587677501927));
#34507=CARTESIAN_POINT('Ctrl Pts',(-83.276340374832,3.94935121612124,-11.4271772949875));
#34508=CARTESIAN_POINT('Ctrl Pts',(-83.2365554066357,5.82359899029299,-10.5954448114821));
#34509=CARTESIAN_POINT('Ctrl Pts',(-83.1967704384394,7.38378811207008,-9.36536998144095));
#34510=CARTESIAN_POINT('Ctrl Pts',(-83.1569854702432,8.9439772338472,-8.13529515139976));
#34511=CARTESIAN_POINT('Ctrl Pts',(-83.117200502047,10.1901077032297,-6.50687797482273));
#34512=CARTESIAN_POINT('Ctrl Pts',(-83.0774155338507,10.9696597020526,-4.67942814989959));
#34513=CARTESIAN_POINT('Ctrl Pts',(-83.0376305656544,11.7492117008756,-2.85197832497647));
#34514=CARTESIAN_POINT('Ctrl Pts',(-82.9978455974581,12.0621852291391,-0.825495851707222));
#34515=CARTESIAN_POINT('Ctrl Pts',(-82.9580606292619,11.8702739778685,1.15198847272976));
#34516=CARTESIAN_POINT('Ctrl Pts',(-82.9182756610656,11.6783627265978,3.12947279716674));
#34517=CARTESIAN_POINT('Ctrl Pts',(-82.8784906928694,10.981566695793,5.05795897277145));
#34518=CARTESIAN_POINT('Ctrl Pts',(-82.8387057246731,9.86517004487055,6.70141043418577));
#34519=CARTESIAN_POINT('Ctrl Pts',(-82.7989207564769,8.74877339394805,8.34486189560009));
#34520=CARTESIAN_POINT('Ctrl Pts',(-82.7591357882806,7.21277612290786,9.70327864282402));
#34521=CARTESIAN_POINT('Ctrl Pts',(-82.7193508200843,5.44517624072831,10.6103976096621));
#34522=CARTESIAN_POINT('Ctrl Pts',(-82.679565851888,3.67757635854875,11.5175165765002));
#34523=CARTESIAN_POINT('Ctrl Pts',(-82.6397808836917,1.67837386522983,11.9733377629524));
#34524=CARTESIAN_POINT('Ctrl Pts',(-82.5999959154955,-0.307739412094615,
11.9220710541212));
#34525=CARTESIAN_POINT('Ctrl Pts',(-82.5602109472993,-2.29385268941909,
11.87080434529));
#34526=CARTESIAN_POINT('Ctrl Pts',(-82.5204259791031,-4.26687675074909,
11.3124497411754));
#34527=CARTESIAN_POINT('Ctrl Pts',(-82.4806410109068,-5.98532373643242,
10.3153469066002));
#34528=CARTESIAN_POINT('Ctrl Pts',(-82.4408560427106,-7.70377072211571,
9.31824407202492));
#34529=CARTESIAN_POINT('Ctrl Pts',(-82.4010710745143,-9.16764063215234,
7.88239300698909));
#34530=CARTESIAN_POINT('Ctrl Pts',(-82.361286106318,-10.1977636774582,6.18353433504965));
#34531=CARTESIAN_POINT('Ctrl Pts',(-82.3215011381217,-11.227886722764,4.48467566311021));
#34532=CARTESIAN_POINT('Ctrl Pts',(-82.2817161699255,-11.8242629033391,
2.52280938426718));
#34533=CARTESIAN_POINT('Ctrl Pts',(-82.2419312017292,-11.9138985183695,
0.538057603617393));
#34534=CARTESIAN_POINT('Ctrl Pts',(-82.2383397502035,-11.9219900660308,
0.358890945100783));
#34535=CARTESIAN_POINT('Ctrl Pts',(-82.2347482986777,-11.9259522069787,
0.179537793630527));
#34536=CARTESIAN_POINT('Ctrl Pts',(-82.2311568471519,-11.9258224962353,
0.000178908662697473));
#34537=CARTESIAN_POINT('Origin',(-92.7728704041008,0.,0.));
#34538=CARTESIAN_POINT('',(-81.5228704041008,-11.0668932874501,4.91862629439992E-5));
#34539=CARTESIAN_POINT('',(-81.425,-11.06595,-4.66420812603649E-14));
#34540=CARTESIAN_POINT('',(-92.7728704041008,-11.06595,-4.66420812603649E-14));
#34541=CARTESIAN_POINT('',(-81.425,-10.149321152349,-4.41097929944913));
#34542=CARTESIAN_POINT('Ctrl Pts',(-81.5228704041008,-11.0668939277106,
4.92196483355134E-5));
#34543=CARTESIAN_POINT('Ctrl Pts',(-81.4902469360672,-11.0665321546601,
-1.51174383270627));
#34544=CARTESIAN_POINT('Ctrl Pts',(-81.4576234680336,-10.7506077524621,
-3.0236872243398));
#34545=CARTESIAN_POINT('Ctrl Pts',(-81.425,-10.149321152349,-4.41097929944913));
#34546=CARTESIAN_POINT('Origin',(-81.425,0.,0.));
#34547=CARTESIAN_POINT('Origin',(-92.7728704041008,0.,0.));
#34548=CARTESIAN_POINT('',(-83.0228704041008,-11.0650302043893,7.38840550997362E-5));
#34549=CARTESIAN_POINT('',(-82.7271295958992,-11.0667132454688,0.000166020487631646));
#34550=CARTESIAN_POINT('',(-92.7728704041008,-11.06595,-4.66420812603649E-14));
#34551=CARTESIAN_POINT('Ctrl Pts',(-83.0228704041008,-11.0650302043893,
7.38840550998376E-5));
#34552=CARTESIAN_POINT('Ctrl Pts',(-83.0012671458212,-11.0647977927194,
-1.00152184229597));
#34553=CARTESIAN_POINT('Ctrl Pts',(-82.9398789193453,-10.6819148380356,
-3.84784936091178));
#34554=CARTESIAN_POINT('Ctrl Pts',(-82.8387057246731,-8.27151795293221,
-8.04356576264067));
#34555=CARTESIAN_POINT('Ctrl Pts',(-82.7193508200843,-3.40317098979375,
-11.0243088802804));
#34556=CARTESIAN_POINT('Ctrl Pts',(-82.5999959154955,2.29823635758004,-11.306417153959));
#34557=CARTESIAN_POINT('Ctrl Pts',(-82.4806410109068,7.43705978076056,-8.82083340892465));
#34558=CARTESIAN_POINT('Ctrl Pts',(-82.361286106318,10.7553688582105,-4.17600247780928));
#34559=CARTESIAN_POINT('Ctrl Pts',(-82.2419312017292,11.4408774690408,1.49107004187632));
#34560=CARTESIAN_POINT('Ctrl Pts',(-82.1225762971404,9.32577815964549,6.79314407704868));
#34561=CARTESIAN_POINT('Ctrl Pts',(-82.0032213925517,4.92782947223121,10.4323283560957));
#34562=CARTESIAN_POINT('Ctrl Pts',(-81.8838664879629,-0.676406317082347,
11.5177874273519));
#34563=CARTESIAN_POINT('Ctrl Pts',(-81.7645115833741,-6.1150519099602,9.78381527403391));
#34564=CARTESIAN_POINT('Ctrl Pts',(-81.6451566787853,-10.0568242125366,
5.65486392012898));
#34565=CARTESIAN_POINT('Ctrl Pts',(-81.5646096190276,-11.0555472977052,
1.93426637659237));
#34566=CARTESIAN_POINT('Ctrl Pts',(-81.5238475274661,-11.0669047633735,
0.0453297616602893));
#34567=CARTESIAN_POINT('Ctrl Pts',(-81.5228704041008,-11.0668939277106,
4.92196483355134E-5));
#34568=CARTESIAN_POINT('',(-81.425,-7.47762833958605,8.15722525234652));
#34569=CARTESIAN_POINT('Origin',(-81.425,0.,0.));
#34570=CARTESIAN_POINT('Ctrl Pts',(-82.7271295958992,-11.0667132454688,
0.000166020487631455));
#34571=CARTESIAN_POINT('Ctrl Pts',(-82.6909360792287,-11.0655002280488,
-1.67714648383287));
#34572=CARTESIAN_POINT('Ctrl Pts',(-82.614957594362,-10.2534263510633,-5.19934407837023));
#34573=CARTESIAN_POINT('Ctrl Pts',(-82.499194141299,-6.66636917491129,-9.416820017226));
#34574=CARTESIAN_POINT('Ctrl Pts',(-82.3798392367102,-1.33616352515641,
-11.4600008190507));
#34575=CARTESIAN_POINT('Ctrl Pts',(-82.2604843321214,4.32110767959995,-10.6978936382306));
#34576=CARTESIAN_POINT('Ctrl Pts',(-82.1411294275327,8.92064463412699,-7.31705529020618));
#34577=CARTESIAN_POINT('Ctrl Pts',(-82.0217745229439,11.3364445890174,-2.14507737917849));
#34578=CARTESIAN_POINT('Ctrl Pts',(-81.9024196183551,10.9773205983354,3.5519900017792));
#34579=CARTESIAN_POINT('Ctrl Pts',(-81.7830647137664,7.93081818705442,8.37957343457652));
#34580=CARTESIAN_POINT('Ctrl Pts',(-81.6637098091775,2.94344912458979,11.155910191377));
#34581=CARTESIAN_POINT('Ctrl Pts',(-81.5443549045888,-2.76549453716151,
11.2014042094999));
#34582=CARTESIAN_POINT('Ctrl Pts',(-81.4647849681962,-6.11821953149998,
9.40337863342461));
#34583=CARTESIAN_POINT('Ctrl Pts',(-81.425,-7.47762833958605,8.15722525234652));
#34584=CARTESIAN_POINT('Origin',(-92.7728704041008,0.,0.));
#34585=CARTESIAN_POINT('',(-84.5228704041007,-11.0666243849915,-0.000196364959975874));
#34586=CARTESIAN_POINT('',(-84.2271295958992,-11.0650096262609,-3.93228210321395E-5));
#34587=CARTESIAN_POINT('',(-92.7728704041008,-11.06595,-4.66420812603649E-14));
#34588=CARTESIAN_POINT('Ctrl Pts',(-84.5228704041008,-11.0666243849915,
-0.000196364959975971));
#34589=CARTESIAN_POINT('Ctrl Pts',(-84.5184717323725,-11.066792356144,-0.204048309631058));
#34590=CARTESIAN_POINT('Ctrl Pts',(-84.474288092448,-11.0113828159013,-2.25160265711946));
#34591=CARTESIAN_POINT('Ctrl Pts',(-84.3903194843273,-9.80445239033203,
-6.08191356265241));
#34592=CARTESIAN_POINT('Ctrl Pts',(-84.2709645797384,-5.68886699611132,
-10.0376168266402));
#34593=CARTESIAN_POINT('Ctrl Pts',(-84.1516096751498,-0.180706798974452,
-11.5362170710623));
#34594=CARTESIAN_POINT('Ctrl Pts',(-84.0322547705609,5.37168852179416,-10.2108727189529));
#34595=CARTESIAN_POINT('Ctrl Pts',(-83.9128998659722,9.60915099398264,-6.38601412721019));
#34596=CARTESIAN_POINT('Ctrl Pts',(-83.7935449613833,11.4943943756167,-0.99792644773947));
#34597=CARTESIAN_POINT('Ctrl Pts',(-83.6741900567946,10.5659309167634,4.63444312957206));
#34598=CARTESIAN_POINT('Ctrl Pts',(-83.5548351522057,7.0510387058728,9.13234977562325));
#34599=CARTESIAN_POINT('Ctrl Pts',(-83.4354802476171,1.81012638584784,11.3947532543155));
#34600=CARTESIAN_POINT('Ctrl Pts',(-83.3161253430282,-3.87388583478548,
10.8678409906937));
#34601=CARTESIAN_POINT('Ctrl Pts',(-83.1967704384395,-8.6096115480947,7.68059556507888));
#34602=CARTESIAN_POINT('Ctrl Pts',(-83.0990187921303,-10.7620932754816,
3.53041677683679));
#34603=CARTESIAN_POINT('Ctrl Pts',(-83.0410521140174,-11.0652258064372,
0.843035751868332));
#34604=CARTESIAN_POINT('Ctrl Pts',(-83.0228704041008,-11.0650302043893,
7.38840550998376E-5));
#34605=CARTESIAN_POINT('Ctrl Pts',(-84.2271295958992,-11.0650096262609,
-3.93228210321395E-5));
#34606=CARTESIAN_POINT('Ctrl Pts',(-84.2081406657801,-11.065118111154,-0.880431154628511));
#34607=CARTESIAN_POINT('Ctrl Pts',(-84.1493667674648,-10.743849849773,-3.60531251949298));
#34608=CARTESIAN_POINT('Ctrl Pts',(-84.0508079009531,-8.53125926061665,
-7.76753330473083));
#34609=CARTESIAN_POINT('Ctrl Pts',(-83.9314529963644,-3.76344689371811,
-10.9065771758865));
#34610=CARTESIAN_POINT('Ctrl Pts',(-83.8120980917756,1.92561768833889,-11.3758056740724));
#34611=CARTESIAN_POINT('Ctrl Pts',(-83.6927431871867,7.1433113126398,-9.06035659838774));
#34612=CARTESIAN_POINT('Ctrl Pts',(-83.573388282598,10.6123974680266,-4.52702752791171));
#34613=CARTESIAN_POINT('Ctrl Pts',(-83.4540333780092,11.4836803397467,1.11447026455969));
#34614=CARTESIAN_POINT('Ctrl Pts',(-83.3346784734204,9.54387907255568,6.48315745825352));
#34615=CARTESIAN_POINT('Ctrl Pts',(-83.2153235688317,5.26783655646332,10.2648358994969));
#34616=CARTESIAN_POINT('Ctrl Pts',(-83.0959686642429,-0.297716860125996,
11.5337904801815));
#34617=CARTESIAN_POINT('Ctrl Pts',(-82.9766137596541,-5.79039248565415,
9.9793944722816));
#34618=CARTESIAN_POINT('Ctrl Pts',(-82.8572588550654,-9.86564059407429,
5.98214765639898));
#34619=CARTESIAN_POINT('Ctrl Pts',(-82.774097467147,-11.0224273794537,2.1767290968266));
#34620=CARTESIAN_POINT('Ctrl Pts',(-82.730721047425,-11.0668336121439,0.166604297477993));
#34621=CARTESIAN_POINT('Ctrl Pts',(-82.7271295958992,-11.0667132454688,
0.000166020487631455));
#34622=CARTESIAN_POINT('Origin',(-92.7728704041008,0.,0.));
#34623=CARTESIAN_POINT('',(-86.0228704041009,-11.065460751515,0.000255221764428716));
#34624=CARTESIAN_POINT('',(-85.7271295958992,-11.0668617871986,-8.70765389315853E-5));
#34625=CARTESIAN_POINT('',(-92.7728704041008,-11.06595,-4.66420812603649E-14));
#34626=CARTESIAN_POINT('Ctrl Pts',(-86.0228704041009,-11.065460751515,0.00025522176442902));
#34627=CARTESIAN_POINT('Ctrl Pts',(-85.9958913507277,-11.064405544315,-1.25044009334015));
#34628=CARTESIAN_POINT('Ctrl Pts',(-85.9291273291583,-10.5406416224597,
-4.34634890493393));
#34629=CARTESIAN_POINT('Ctrl Pts',(-85.8225783393926,-7.7096875531033,-8.58357018328625));
#34630=CARTESIAN_POINT('Ctrl Pts',(-85.7032234348039,-2.65123622795373,
-11.2288871096588));
#34631=CARTESIAN_POINT('Ctrl Pts',(-85.583868530215,3.05620983905482,-11.1254905814324));
#34632=CARTESIAN_POINT('Ctrl Pts',(-85.4645136256263,8.01552788387837,-8.29869098115147));
#34633=CARTESIAN_POINT('Ctrl Pts',(-85.3451587210375,11.0127290131994,-3.44045911757623));
#34634=CARTESIAN_POINT('Ctrl Pts',(-85.2258038164487,11.3141299162988,2.25996094988123));
#34635=CARTESIAN_POINT('Ctrl Pts',(-85.10644891186,8.84595082235115,7.40716634796478));
#34636=CARTESIAN_POINT('Ctrl Pts',(-84.9870940072712,4.21237601227739,10.7411753355518));
#34637=CARTESIAN_POINT('Ctrl Pts',(-84.8677391026824,-1.45234413817624,
11.4458575808972));
#34638=CARTESIAN_POINT('Ctrl Pts',(-84.7483841980936,-6.7615457199306,9.34871428246502));
#34639=CARTESIAN_POINT('Ctrl Pts',(-84.6334279652331,-10.2809268459538,
5.1247300936646));
#34640=CARTESIAN_POINT('Ctrl Pts',(-84.5582567005688,-11.0652730959279,
1.63974537094761));
#34641=CARTESIAN_POINT('Ctrl Pts',(-84.5228704041008,-11.0666243849915,
-0.000196364959975971));
#34642=CARTESIAN_POINT('Ctrl Pts',(-85.7271295958992,-11.0668617871986,
-8.70765389308394E-5));
#34643=CARTESIAN_POINT('Ctrl Pts',(-85.7253452523315,-11.0668963362517,
-0.0827755069023009));
#34644=CARTESIAN_POINT('Ctrl Pts',(-85.6837759405676,-11.045758910777,-2.00912511781817));
#34645=CARTESIAN_POINT('Ctrl Pts',(-85.6024216606073,-9.99893271614051,
-5.75658776984223));
#34646=CARTESIAN_POINT('Ctrl Pts',(-85.4830667560185,-6.01549992917226,
-9.84533995430987));
#34647=CARTESIAN_POINT('Ctrl Pts',(-85.3637118514298,-0.559536032933944,
-11.5240564751155));
#34648=CARTESIAN_POINT('Ctrl Pts',(-85.2443569468409,5.03339639874698,-10.3818051853656));
#34649=CARTESIAN_POINT('Ctrl Pts',(-85.1250020422522,9.39420633525482,-6.69819718614323));
#34650=CARTESIAN_POINT('Ctrl Pts',(-85.0056471376634,11.4554133728453,-1.37494097002217));
#34651=CARTESIAN_POINT('Ctrl Pts',(-84.8862922330746,10.7124557092996,4.28488633339115));
#34652=CARTESIAN_POINT('Ctrl Pts',(-84.7669373284858,7.34720156593731,8.89581853250784));
#34653=CARTESIAN_POINT('Ctrl Pts',(-84.647582423897,2.18342975997975,11.3291479245805));
#34654=CARTESIAN_POINT('Ctrl Pts',(-84.5282275193083,-3.5148226850366,10.9892210691436));
#34655=CARTESIAN_POINT('Ctrl Pts',(-84.4088726147195,-8.35268350706726,
7.95924848492489));
#34656=CARTESIAN_POINT('Ctrl Pts',(-84.3085066402497,-10.7015054577232,
3.77296701935926));
#34657=CARTESIAN_POINT('Ctrl Pts',(-84.2479256339763,-11.0648908172521,
0.964136222734465));
#34658=CARTESIAN_POINT('Ctrl Pts',(-84.2271295958992,-11.0650096262609,
-3.93228210321395E-5));
#34659=CARTESIAN_POINT('Origin',(-92.7728704041008,0.,0.));
#34660=CARTESIAN_POINT('',(-87.5228704041008,-11.0658700602947,-0.000290735752023665));
#34661=CARTESIAN_POINT('',(-87.2271295958992,-11.065192145401,0.000181283075004757));
#34662=CARTESIAN_POINT('',(-92.7728704041008,-11.06595,-4.66420812603649E-14));
#34663=CARTESIAN_POINT('Ctrl Pts',(-87.5228704041008,-11.0658700602947,
-0.000290735752023694));
#34664=CARTESIAN_POINT('Ctrl Pts',(-87.513095937279,-11.0663323771202,-0.453367480613647));
#34665=CARTESIAN_POINT('Ctrl Pts',(-87.4635365022611,-10.9279235443852,
-2.75031985271847));
#34666=CARTESIAN_POINT('Ctrl Pts',(-87.3741920990468,-9.37154264007224,
-6.72986982053519));
#34667=CARTESIAN_POINT('Ctrl Pts',(-87.2548371944581,-4.99832326681662,
-10.398736643432));
#34668=CARTESIAN_POINT('Ctrl Pts',(-87.1354822898692,0.598433067870375,
-11.5221021137892));
#34669=CARTESIAN_POINT('Ctrl Pts',(-87.0161273852805,6.04869928207646,-9.82497818079478));
#34670=CARTESIAN_POINT('Ctrl Pts',(-86.8967724806917,10.0183075346351,-5.72280293206974));
#34671=CARTESIAN_POINT('Ctrl Pts',(-86.7774175761028,11.5355394792043,-0.219745720288259));
#34672=CARTESIAN_POINT('Ctrl Pts',(-86.6580626715142,10.2289926946021,5.33710293246003));
#34673=CARTESIAN_POINT('Ctrl Pts',(-86.5387077669253,6.41849609092341,9.58748492508142));
#34674=CARTESIAN_POINT('Ctrl Pts',(-86.4193528623365,1.03681915645036,11.4909514529782));
#34675=CARTESIAN_POINT('Ctrl Pts',(-86.2999979577478,-4.59866020185083,
10.5815539315257));
#34676=CARTESIAN_POINT('Ctrl Pts',(-86.1806430531589,-9.10843591325322,
7.08190330857717));
#34677=CARTESIAN_POINT('Ctrl Pts',(-86.0882672019434,-10.8731611950013,
3.03159876678569));
#34678=CARTESIAN_POINT('Ctrl Pts',(-86.035676318924,-11.0659616176254,0.593911991459538));
#34679=CARTESIAN_POINT('Ctrl Pts',(-86.0228704041009,-11.065460751515,0.00025522176442902));
#34680=CARTESIAN_POINT('Ctrl Pts',(-87.2271295958992,-11.065192145401,0.000181283075005034));
#34681=CARTESIAN_POINT('Ctrl Pts',(-87.2027648706866,-11.0645372281205,
-1.12939750798797));
#34682=CARTESIAN_POINT('Ctrl Pts',(-87.1386151772778,-10.6117081325261,
-4.10396985076007));
#34683=CARTESIAN_POINT('Ctrl Pts',(-87.0346805156727,-7.98746940186916,
-8.32570061724489));
#34684=CARTESIAN_POINT('Ctrl Pts',(-86.9153256110839,-3.01863758058317,
-11.1357435930835));
#34685=CARTESIAN_POINT('Ctrl Pts',(-86.7959707064951,2.68912496921423,-11.2198736674593));
#34686=CARTESIAN_POINT('Ctrl Pts',(-86.6766158019064,7.73861801182051,-8.55749668308028));
#34687=CARTESIAN_POINT('Ctrl Pts',(-86.5572608973175,10.8937787629573,-3.80033452179447));
#34688=CARTESIAN_POINT('Ctrl Pts',(-86.4379059927288,11.3822570579663,1.88710955701514));
#34689=CARTESIAN_POINT('Ctrl Pts',(-86.31855108814,9.08447854823605,7.11260906562713));
#34690=CARTESIAN_POINT('Ctrl Pts',(-86.1991961835512,4.56291524401145,10.5970166881896));
#34691=CARTESIAN_POINT('Ctrl Pts',(-86.0798412789624,-1.07560171741225,
11.4873860890675));
#34692=CARTESIAN_POINT('Ctrl Pts',(-85.9604863743737,-6.45082269201481,
9.56576420418091));
#34693=CARTESIAN_POINT('Ctrl Pts',(-85.8429158133526,-10.1901984085959,
5.36627856497651));
#34694=CARTESIAN_POINT('Ctrl Pts',(-85.7651302205278,-11.0661260064756,
1.7609033852933));
#34695=CARTESIAN_POINT('Ctrl Pts',(-85.7271295958992,-11.0668617871986,
-8.70765389308394E-5));
#34696=CARTESIAN_POINT('Origin',(-92.7728704041008,0.,0.));
#34697=CARTESIAN_POINT('',(-89.0228704041008,-11.0662155972561,0.000275354078309783));
#34698=CARTESIAN_POINT('',(-88.7271295958992,-11.0662550916496,-0.000269981886922288));
#34699=CARTESIAN_POINT('',(-92.7728704041008,-11.06595,-4.66420812603649E-14));
#34700=CARTESIAN_POINT('Ctrl Pts',(-89.0228704041008,-11.0662155972561,
0.000275354078309552));
#34701=CARTESIAN_POINT('Ctrl Pts',(-88.9905155556342,-11.0646746332228,
-1.49933692734806));
#34702=CARTESIAN_POINT('Ctrl Pts',(-88.9183757389713,-10.3801459586505,
-4.84430558557994));
#34703=CARTESIAN_POINT('Ctrl Pts',(-88.8064509541122,-7.11268667591289,
-9.08441704154723));
#34704=CARTESIAN_POINT('Ctrl Pts',(-88.6870960495234,-1.88720699773628,
-11.3822412941864));
#34705=CARTESIAN_POINT('Ctrl Pts',(-88.5677411449346,3.80024137539898,-10.8938111540241));
#34706=CARTESIAN_POINT('Ctrl Pts',(-88.4483862403457,8.55743050117986,-7.73869132528777));
#34707=CARTESIAN_POINT('Ctrl Pts',(-88.3290313357571,11.2198507137954,-2.6892209233878));
#34708=CARTESIAN_POINT('Ctrl Pts',(-88.2096764311682,11.1357694560897,3.01854231284303));
#34709=CARTESIAN_POINT('Ctrl Pts',(-88.0903215265796,8.32576898055664,7.9873982188198));
#34710=CARTESIAN_POINT('Ctrl Pts',(-87.9709666219907,3.47770782525073,11.0010230180077));
#34711=CARTESIAN_POINT('Ctrl Pts',(-87.8516117174019,-2.22165962238982,
11.3217131134804));
#34712=CARTESIAN_POINT('Ctrl Pts',(-87.7322568128132,-7.37718816438983,
8.87096691632776));
#34713=CARTESIAN_POINT('Ctrl Pts',(-87.6226763750461,-10.4525402687832,
4.62723777833816));
#34714=CARTESIAN_POINT('Ctrl Pts',(-87.5528809054753,-11.0644506110316,
1.39078874944263));
#34715=CARTESIAN_POINT('Ctrl Pts',(-87.5228704041008,-11.0658700602947,
-0.000290735752023694));
#34716=CARTESIAN_POINT('Ctrl Pts',(-88.7271295958992,-11.0662550916496,
-0.000269981886922149));
#34717=CARTESIAN_POINT('Ctrl Pts',(-88.719969457238,-11.0665935271679,-0.332131280800377));
#34718=CARTESIAN_POINT('Ctrl Pts',(-88.6730243503806,-10.9706735787383,
-2.50776908882701));
#34719=CARTESIAN_POINT('Ctrl Pts',(-88.5862942753268,-9.58753979769892,
-6.41841405704041));
#34720=CARTESIAN_POINT('Ctrl Pts',(-88.4669393707381,-5.33719041442222,
-10.2289469935215));
#34721=CARTESIAN_POINT('Ctrl Pts',(-88.3475844661493,0.219647037160976,
-11.5355413152965));
#34722=CARTESIAN_POINT('Ctrl Pts',(-88.2282295615605,5.72271720750059,-10.0183564501475));
#34723=CARTESIAN_POINT('Ctrl Pts',(-88.1088746569716,9.82492639772949,-6.0487833070047));
#34724=CARTESIAN_POINT('Ctrl Pts',(-87.989519752383,11.5220969489527,-0.598531631862895));
#34725=CARTESIAN_POINT('Ctrl Pts',(-87.8701648477941,10.3987793606657,4.99823429024215));
#34726=CARTESIAN_POINT('Ctrl Pts',(-87.7508099432054,6.72994996350157,9.37148503193342));
#34727=CARTESIAN_POINT('Ctrl Pts',(-87.6314550386166,1.41369960344878,11.4506948105535));
#34728=CARTESIAN_POINT('Ctrl Pts',(-87.5121001340278,-4.24860954964163,
10.7268949425594));
#34729=CARTESIAN_POINT('Ctrl Pts',(-87.3927452294391,-8.87090377354262,
7.37726402227169));
#34730=CARTESIAN_POINT('Ctrl Pts',(-87.2977550500628,-10.8213976376337,
3.27418514836392));
#34731=CARTESIAN_POINT('Ctrl Pts',(-87.2425498388829,-11.0656066373975,
0.715082816969709));
#34732=CARTESIAN_POINT('Ctrl Pts',(-87.2271295958992,-11.065192145401,0.000181283075005034));
#34733=CARTESIAN_POINT('Origin',(-90.25,0.,0.));
#34734=CARTESIAN_POINT('',(-90.,15.5,-1.8982025386784E-15));
#34735=CARTESIAN_POINT('Origin',(-90.,0.,0.));
#34736=CARTESIAN_POINT('',(-90.5,16.,1.95943487863577E-15));
#34737=CARTESIAN_POINT('',(-90.25,15.75,1.92881870865708E-15));
#34738=CARTESIAN_POINT('',(-90.5,-16.,-1.95943487863577E-15));
#34739=CARTESIAN_POINT('Origin',(-90.5,0.,0.));
#34740=CARTESIAN_POINT('Origin',(-90.5,0.,0.));
#34741=CARTESIAN_POINT('Origin',(-91.5,0.,0.));
#34742=CARTESIAN_POINT('',(-92.5,-16.,-1.95943487863577E-15));
#34743=CARTESIAN_POINT('',(-91.5,-16.,-1.95943487863577E-15));
#34744=CARTESIAN_POINT('',(-92.5,16.,-1.95943487863577E-15));
#34745=CARTESIAN_POINT('Origin',(-92.5,0.,0.));
#34746=CARTESIAN_POINT('Origin',(-92.5,0.,0.));
#34747=CARTESIAN_POINT('Origin',(-90.,12.,0.));
#34748=CARTESIAN_POINT('',(-90.,6.42428395783992,-9.0102067141404));
#34749=CARTESIAN_POINT('Ctrl Pts',(-90.,5.13009691060825,10.7656670051306));
#34750=CARTESIAN_POINT('Ctrl Pts',(-90.,5.38142570207304,10.63534500805));
#34751=CARTESIAN_POINT('Ctrl Pts',(-90.,5.62776587470053,10.496194090036));
#34752=CARTESIAN_POINT('Ctrl Pts',(-90.,5.86860373811413,10.3483657837986));
#34753=CARTESIAN_POINT('Ctrl Pts',(-90.,5.89059422220645,10.334867839702));
#34754=CARTESIAN_POINT('Ctrl Pts',(-90.,5.91253881540746,10.321297518862));
#34755=CARTESIAN_POINT('Ctrl Pts',(-90.,5.93443711591287,10.3076549177303));
#34756=CARTESIAN_POINT('Ctrl Pts',(-90.,6.17470730136342,10.1579670319908));
#34757=CARTESIAN_POINT('Ctrl Pts',(-90.,6.4094071003827,9.99958102185828));
#34758=CARTESIAN_POINT('Ctrl Pts',(-90.,6.63816875447367,9.83291388620034));
#34759=CARTESIAN_POINT('Ctrl Pts',(-90.,6.86708098763998,9.66613704429256));
#34760=CARTESIAN_POINT('Ctrl Pts',(-90.,7.09004769008821,9.49106769853988));
#34761=CARTESIAN_POINT('Ctrl Pts',(-90.,7.30666447004526,9.30808587696727));
#34762=CARTESIAN_POINT('Ctrl Pts',(-90.,7.37724818810362,9.24846197661085));
#34763=CARTESIAN_POINT('Ctrl Pts',(-90.,7.44715738756786,9.18799769541298));
#34764=CARTESIAN_POINT('Ctrl Pts',(-90.,7.51637713519723,9.12670544422352));
#34765=CARTESIAN_POINT('Ctrl Pts',(-90.,7.5638011805984,9.08471270945205));
#34766=CARTESIAN_POINT('Ctrl Pts',(-90.,7.61090159178926,9.04233132367685));
#34767=CARTESIAN_POINT('Ctrl Pts',(-90.,7.65767343085564,8.99956519068863));
#34768=CARTESIAN_POINT('Ctrl Pts',(-90.,7.68556498060487,8.97406237212017));
#34769=CARTESIAN_POINT('Ctrl Pts',(-90.,7.71333301047639,8.94842881556734));
#34770=CARTESIAN_POINT('Ctrl Pts',(-90.,7.74097359853661,8.922668405457));
#34771=CARTESIAN_POINT('Ctrl Pts',(-90.,7.94709453709131,8.73056829897841));
#34772=CARTESIAN_POINT('Ctrl Pts',(-90.,8.14618697943012,8.53136626644155));
#34773=CARTESIAN_POINT('Ctrl Pts',(-90.,8.33789206599765,8.32547463222084));
#34774=CARTESIAN_POINT('Ctrl Pts',(-90.,8.52924341455732,8.1199629133056));
#34775=CARTESIAN_POINT('Ctrl Pts',(-90.,8.71323504729152,7.90778577042483));
#34776=CARTESIAN_POINT('Ctrl Pts',(-90.,8.88947131067135,7.68931924303648));
#34777=CARTESIAN_POINT('Ctrl Pts',(-90.,9.06438024748662,7.47249810020014));
#34778=CARTESIAN_POINT('Ctrl Pts',(-90.,9.2316505465745,7.24948146658954));
#34779=CARTESIAN_POINT('Ctrl Pts',(-90.,9.39085163563897,7.02061071827486));
#34780=CARTESIAN_POINT('Ctrl Pts',(-90.,9.4429730085429,6.94567996440997));
#34781=CARTESIAN_POINT('Ctrl Pts',(-90.,9.4942290980679,6.87012154957565));
#34782=CARTESIAN_POINT('Ctrl Pts',(-90.,9.54460366504352,6.79394696955633));
#34783=CARTESIAN_POINT('Ctrl Pts',(-90.,9.56885339937438,6.75727740713355));
#34784=CARTESIAN_POINT('Ctrl Pts',(-90.,9.59289884560302,6.72046505461935));
#34785=CARTESIAN_POINT('Ctrl Pts',(-90.,9.61673814334246,6.6835111777183));
#34786=CARTESIAN_POINT('Ctrl Pts',(-90.,9.63482522819697,6.65547394631501));
#34787=CARTESIAN_POINT('Ctrl Pts',(-90.,9.65279406781826,6.62735450526691));
#34788=CARTESIAN_POINT('Ctrl Pts',(-90.,9.67063513222111,6.59916738127204));
#34789=CARTESIAN_POINT('Ctrl Pts',(-90.,9.77582411073673,6.43297915878919));
#34790=CARTESIAN_POINT('Ctrl Pts',(-90.,9.87664553414384,6.26432609926212));
#34791=CARTESIAN_POINT('Ctrl Pts',(-90.,9.97297960718523,6.09334570164801));
#34792=CARTESIAN_POINT('Ctrl Pts',(-90.,10.1090715536707,5.85180027138097));
#34793=CARTESIAN_POINT('Ctrl Pts',(-90.,10.2362100229841,5.60561105936211));
#34794=CARTESIAN_POINT('Ctrl Pts',(-90.,10.3543191903964,5.35532203303746));
#34795=CARTESIAN_POINT('Ctrl Pts',(-90.,10.4732217365238,5.10335173174952));
#34796=CARTESIAN_POINT('Ctrl Pts',(-90.,10.5829734569656,4.84722574878759));
#34797=CARTESIAN_POINT('Ctrl Pts',(-90.,10.6834490166989,4.58747640854734));
#34798=CARTESIAN_POINT('Ctrl Pts',(-90.,10.7839018241246,4.32778588755518));
#34799=CARTESIAN_POINT('Ctrl Pts',(-90.,10.8750828153631,4.06447302517473));
#34800=CARTESIAN_POINT('Ctrl Pts',(-90.,10.9568165288933,3.79805645882746));
#34801=CARTESIAN_POINT('Ctrl Pts',(-90.,11.0372022543992,3.53603375060076));
#34802=CARTESIAN_POINT('Ctrl Pts',(-90.,11.1084497580427,3.27100827338904));
#34803=CARTESIAN_POINT('Ctrl Pts',(-90.,11.1703426294259,3.00346961322391));
#34804=CARTESIAN_POINT('Ctrl Pts',(-90.,11.1935524561946,2.90314261566199));
#34805=CARTESIAN_POINT('Ctrl Pts',(-90.,11.2154462823607,2.80246220808664));
#34806=CARTESIAN_POINT('Ctrl Pts',(-90.,11.2360108513013,2.70145432537238));
#34807=CARTESIAN_POINT('Ctrl Pts',(-90.,11.2500737341414,2.63238105548534));
#34808=CARTESIAN_POINT('Ctrl Pts',(-90.,11.2635149851746,2.56315464787577));
#34809=CARTESIAN_POINT('Ctrl Pts',(-90.,11.2763300877809,2.49378343749949));
#34810=CARTESIAN_POINT('Ctrl Pts',(-90.,11.281580840756,2.46535985787929));
#34811=CARTESIAN_POINT('Ctrl Pts',(-90.,11.2867263799758,2.43691228547538));
#34812=CARTESIAN_POINT('Ctrl Pts',(-90.,11.2917640894315,2.40845488838702));
#34813=CARTESIAN_POINT('Ctrl Pts',(-90.,11.3399768555613,2.13610694086531));
#34814=CARTESIAN_POINT('Ctrl Pts',(-90.,11.3783768067611,1.86254282314492));
#34815=CARTESIAN_POINT('Ctrl Pts',(-90.,11.4068617806356,1.58827966874211));
#34816=CARTESIAN_POINT('Ctrl Pts',(-90.,11.4352887946213,1.31457457214283));
#34817=CARTESIAN_POINT('Ctrl Pts',(-90.,11.4538412446679,1.04017266307592));
#34818=CARTESIAN_POINT('Ctrl Pts',(-90.,11.4623666776379,0.765579031056406));
#34819=CARTESIAN_POINT('Ctrl Pts',(-90.,11.4645277885494,0.695972326451475));
#34820=CARTESIAN_POINT('Ctrl Pts',(-90.,11.4660443321508,0.626353283748583));
#34821=CARTESIAN_POINT('Ctrl Pts',(-90.,11.4669132910905,0.556730111859395));
#34822=CARTESIAN_POINT('Ctrl Pts',(-90.,11.4703524607466,0.281175204517033));
#34823=CARTESIAN_POINT('Ctrl Pts',(-90.,11.4636517873567,0.0055550935556139));
#34824=CARTESIAN_POINT('Ctrl Pts',(-90.,11.4469479467724,-0.269598067443254));
#34825=CARTESIAN_POINT('Ctrl Pts',(-90.,11.4302653802983,-0.544400791748682));
#34826=CARTESIAN_POINT('Ctrl Pts',(-90.,11.4036049324252,-0.818738377219698));
#34827=CARTESIAN_POINT('Ctrl Pts',(-90.,11.3670523229692,-1.09206872465835));
#34828=CARTESIAN_POINT('Ctrl Pts',(-90.,11.3447418592934,-1.25890022803875));
#34829=CARTESIAN_POINT('Ctrl Pts',(-90.,11.3187451354215,-1.42535621584432));
#34830=CARTESIAN_POINT('Ctrl Pts',(-90.,11.2890728104253,-1.59130971323021));
#34831=CARTESIAN_POINT('Ctrl Pts',(-90.,11.2760911682395,-1.66391436833653));
#34832=CARTESIAN_POINT('Ctrl Pts',(-90.,11.2624059083653,-1.73642280066201));
#34833=CARTESIAN_POINT('Ctrl Pts',(-90.,11.24801753262,-1.8088241590467));
#34834=CARTESIAN_POINT('Ctrl Pts',(-90.,11.2386133705796,-1.85614528258763));
#34835=CARTESIAN_POINT('Ctrl Pts',(-90.,11.2289088427027,-1.90342066283882));
#34836=CARTESIAN_POINT('Ctrl Pts',(-90.,11.2189040351068,-1.95064723561348));
#34837=CARTESIAN_POINT('Ctrl Pts',(-90.,11.2135629399335,-1.97585927667222));
#34838=CARTESIAN_POINT('Ctrl Pts',(-90.,11.2081367261043,-2.00105513468646));
#34839=CARTESIAN_POINT('Ctrl Pts',(-90.,11.2026273691943,-2.02622584437508));
#34840=CARTESIAN_POINT('Ctrl Pts',(-90.,11.1440984837332,-2.29362794019419));
#34841=CARTESIAN_POINT('Ctrl Pts',(-90.,11.0761321356989,-2.55846899415871));
#34842=CARTESIAN_POINT('Ctrl Pts',(-90.,10.9989076859169,-2.82024219140262));
#34843=CARTESIAN_POINT('Ctrl Pts',(-90.,10.9216242802013,-3.0822152357584));
#34844=CARTESIAN_POINT('Ctrl Pts',(-90.,10.8350684457149,-3.34111635466465));
#34845=CARTESIAN_POINT('Ctrl Pts',(-90.,10.7393689679669,-3.59642631329222));
#34846=CARTESIAN_POINT('Ctrl Pts',(-90.,10.6445416932764,-3.84940938224622));
#34847=CARTESIAN_POINT('Ctrl Pts',(-90.,10.5407364399718,-4.0988670139967));
#34848=CARTESIAN_POINT('Ctrl Pts',(-90.,10.4280318007549,-4.34427424590613));
#34849=CARTESIAN_POINT('Ctrl Pts',(-90.,10.3389543367021,-4.53823479651512));
#34850=CARTESIAN_POINT('Ctrl Pts',(-90.,10.2443167396394,-4.72966489136653));
#34851=CARTESIAN_POINT('Ctrl Pts',(-90.,10.1441383060101,-4.91829300030524));
#34852=CARTESIAN_POINT('Ctrl Pts',(-90.,10.0350500930934,-5.12369752266081));
#34853=CARTESIAN_POINT('Ctrl Pts',(-90.,9.91939159180428,-5.32577984787966));
#34854=CARTESIAN_POINT('Ctrl Pts',(-90.,9.79736644993105,-5.52427284227006));
#34855=CARTESIAN_POINT('Ctrl Pts',(-90.,9.74398045036152,-5.61111352731585));
#34856=CARTESIAN_POINT('Ctrl Pts',(-90.,9.68937558727447,-5.69726693803969));
#34857=CARTESIAN_POINT('Ctrl Pts',(-90.,9.63356781953306,-5.78270944804998));
#34858=CARTESIAN_POINT('Ctrl Pts',(-90.,9.5976005282019,-5.83777589800808));
#34859=CARTESIAN_POINT('Ctrl Pts',(-90.,9.56113358369664,-5.89254705121343));
#34860=CARTESIAN_POINT('Ctrl Pts',(-90.,9.5241711249039,-5.94701640003021));
#34861=CARTESIAN_POINT('Ctrl Pts',(-90.,9.50389726234252,-5.9768927699414));
#34862=CARTESIAN_POINT('Ctrl Pts',(-90.,9.4834724625547,-6.00668093496707));
#34863=CARTESIAN_POINT('Ctrl Pts',(-90.,9.46291188231344,-6.03635915674249));
#34864=CARTESIAN_POINT('Ctrl Pts',(-90.,9.30976555255365,-6.25741861544314));
#34865=CARTESIAN_POINT('Ctrl Pts',(-90.,9.14893478031223,-6.47261211276324));
#34866=CARTESIAN_POINT('Ctrl Pts',(-90.,8.98082954059386,-6.68160127162625));
#34867=CARTESIAN_POINT('Ctrl Pts',(-90.,8.81151510059202,-6.89209371349556));
#34868=CARTESIAN_POINT('Ctrl Pts',(-90.,8.63482075206015,-7.09629271941038));
#34869=CARTESIAN_POINT('Ctrl Pts',(-90.,8.45112207888021,-7.2938225125168));
#34870=CARTESIAN_POINT('Ctrl Pts',(-90.,8.26780812280964,-7.49093862222691));
#34871=CARTESIAN_POINT('Ctrl Pts',(-90.,8.07751868545223,-7.6814138584871));
#34872=CARTESIAN_POINT('Ctrl Pts',(-90.,7.88059071023121,-7.86483819093346));
#34873=CARTESIAN_POINT('Ctrl Pts',(-90.,7.68518613482991,-8.04684358534082));
#34874=CARTESIAN_POINT('Ctrl Pts',(-90.,7.48324486788944,-8.22190712647571));
#34875=CARTESIAN_POINT('Ctrl Pts',(-90.,7.27506729716046,-8.38958611218002));
#34876=CARTESIAN_POINT('Ctrl Pts',(-90.,7.07054495646357,-8.55432095139367));
#34877=CARTESIAN_POINT('Ctrl Pts',(-90.,6.86000293117097,-8.71192855691827));
#34878=CARTESIAN_POINT('Ctrl Pts',(-90.,6.6437050061379,-8.86194356787701));
#34879=CARTESIAN_POINT('Ctrl Pts',(-90.,6.57120824497411,-8.91222422784541));
#34880=CARTESIAN_POINT('Ctrl Pts',(-90.,6.49806472103886,-8.96165153702105));
#34881=CARTESIAN_POINT('Ctrl Pts',(-90.,6.42428395783973,-9.01020671414053));
#34882=CARTESIAN_POINT('',(-90.,-6.42475130859185,-9.01043996637154));
#34883=CARTESIAN_POINT('Origin',(-90.,0.,0.));
#34884=CARTESIAN_POINT('Ctrl Pts',(-90.,-6.42475130859154,-9.01043996637175));
#34885=CARTESIAN_POINT('Ctrl Pts',(-90.,-6.65061596671456,-8.86211493166386));
#34886=CARTESIAN_POINT('Ctrl Pts',(-89.9999999999999,-6.87072984044529,
-8.70566715326926));
#34887=CARTESIAN_POINT('Ctrl Pts',(-89.9999999999999,-7.08460872649498,
-8.54135125534634));
#34888=CARTESIAN_POINT('Ctrl Pts',(-89.9999999999999,-7.09832383863764,
-8.53081439961243));
#34889=CARTESIAN_POINT('Ctrl Pts',(-89.9999999999999,-7.11201330530386,
-8.52024517293795));
#34890=CARTESIAN_POINT('Ctrl Pts',(-89.9999999999999,-7.12567699593402,
-8.50964363574394));
#34891=CARTESIAN_POINT('Ctrl Pts',(-89.9999999999999,-7.33729564816288,
-8.34545058766665));
#34892=CARTESIAN_POINT('Ctrl Pts',(-90.,-7.54273377508571,-8.17351106236173));
#34893=CARTESIAN_POINT('Ctrl Pts',(-90.,-7.74171723733581,-7.9942942910195));
#34894=CARTESIAN_POINT('Ctrl Pts',(-90.,-7.94191952622316,-7.81397976927991));
#34895=CARTESIAN_POINT('Ctrl Pts',(-89.9999999999999,-8.13558827492983,
-7.62629814154647));
#34896=CARTESIAN_POINT('Ctrl Pts',(-89.9999999999999,-8.32241215048194,
-7.43168519135534));
#34897=CARTESIAN_POINT('Ctrl Pts',(-89.9999999999999,-8.38001350953885,
-7.37168231223749));
#34898=CARTESIAN_POINT('Ctrl Pts',(-89.9999999999999,-8.43696393552139,
-7.31102026254922));
#34899=CARTESIAN_POINT('Ctrl Pts',(-89.9999999999999,-8.49325359145673,
-7.24971111436292));
#34900=CARTESIAN_POINT('Ctrl Pts',(-89.9999999999999,-8.52511339921065,
-7.21501028625668));
#34901=CARTESIAN_POINT('Ctrl Pts',(-89.9999999999999,-8.5567615207414,-7.18010215242168));
#34902=CARTESIAN_POINT('Ctrl Pts',(-89.9999999999999,-8.58819612090012,
-7.14498885930322));
#34903=CARTESIAN_POINT('Ctrl Pts',(-89.9999999999999,-8.61211097529082,
-7.11827532428557));
#34904=CARTESIAN_POINT('Ctrl Pts',(-90.,-8.63590251481974,-7.09144266968923));
#34905=CARTESIAN_POINT('Ctrl Pts',(-90.,-8.65955976364048,-7.06450359547617));
#34906=CARTESIAN_POINT('Ctrl Pts',(-90.,-8.83805698972194,-6.8612445412781));
#34907=CARTESIAN_POINT('Ctrl Pts',(-90.,-9.00905478459883,-6.6517718956029));
#34908=CARTESIAN_POINT('Ctrl Pts',(-90.,-9.17227989292783,-6.4365623541276));
#34909=CARTESIAN_POINT('Ctrl Pts',(-90.,-9.33663083357885,-6.2198684217992));
#34910=CARTESIAN_POINT('Ctrl Pts',(-90.,-9.49310194101511,-5.99735772885397));
#34911=CARTESIAN_POINT('Ctrl Pts',(-90.,-9.64137918380223,-5.76947781861025));
#34912=CARTESIAN_POINT('Ctrl Pts',(-90.,-9.78920952329607,-5.54228473178221));
#34913=CARTESIAN_POINT('Ctrl Pts',(-90.,-9.9288957109934,-5.30975423589191));
#34914=CARTESIAN_POINT('Ctrl Pts',(-90.,-10.0600855719573,-5.07229842674199));
#34915=CARTESIAN_POINT('Ctrl Pts',(-90.,-10.1025381524142,-4.99545855688614));
#34916=CARTESIAN_POINT('Ctrl Pts',(-90.,-10.1441006967004,-4.9181027202424));
#34917=CARTESIAN_POINT('Ctrl Pts',(-90.,-10.184760241468,-4.8402443089206));
#34918=CARTESIAN_POINT('Ctrl Pts',(-90.,-10.2071957271072,-4.79728290148023));
#34919=CARTESIAN_POINT('Ctrl Pts',(-90.,-10.2293562663178,-4.7541684701326));
#34920=CARTESIAN_POINT('Ctrl Pts',(-90.,-10.2512396111472,-4.71090323342713));
#34921=CARTESIAN_POINT('Ctrl Pts',(-90.,-10.2652344513955,-4.68323424220498));
#34922=CARTESIAN_POINT('Ctrl Pts',(-90.,-10.2791136353224,-4.65550804712252));
#34923=CARTESIAN_POINT('Ctrl Pts',(-90.,-10.2928733408437,-4.62773215676248));
#34924=CARTESIAN_POINT('Ctrl Pts',(-90.,-10.3745756942675,-4.46280452750792));
#34925=CARTESIAN_POINT('Ctrl Pts',(-90.,-10.4521032429591,-4.29605217209308));
#34926=CARTESIAN_POINT('Ctrl Pts',(-90.,-10.5253730189402,-4.12761863166149));
#34927=CARTESIAN_POINT('Ctrl Pts',(-90.,-10.633017677609,-3.8801636514142));
#34928=CARTESIAN_POINT('Ctrl Pts',(-90.,-10.7314745633192,-3.62908127751788));
#34929=CARTESIAN_POINT('Ctrl Pts',(-90.,-10.820768106391,-3.37492377019595));
#34930=CARTESIAN_POINT('Ctrl Pts',(-90.,-10.911052892199,-3.11794487429105));
#34931=CARTESIAN_POINT('Ctrl Pts',(-90.,-10.9919699583455,-2.85782164311628));
#34932=CARTESIAN_POINT('Ctrl Pts',(-90.,-11.0634983479278,-2.59509741224024));
#34933=CARTESIAN_POINT('Ctrl Pts',(-90.,-11.135398801024,-2.33100658970638));
#34934=CARTESIAN_POINT('Ctrl Pts',(-90.,-11.1978128183106,-2.06428703600773));
#34935=CARTESIAN_POINT('Ctrl Pts',(-90.,-11.2506700006432,-1.7954717017297));
#34936=CARTESIAN_POINT('Ctrl Pts',(-90.,-11.3030143363181,-1.52926454744956));
#34937=CARTESIAN_POINT('Ctrl Pts',(-90.,-11.34598643978,-1.26100146289971));
#34938=CARTESIAN_POINT('Ctrl Pts',(-90.,-11.3794684511118,-0.991190731214159));
#34939=CARTESIAN_POINT('Ctrl Pts',(-90.,-11.3920242053612,-0.890011706832077));
#34940=CARTESIAN_POINT('Ctrl Pts',(-90.,-11.4032449091829,-0.788614997625171));
#34941=CARTESIAN_POINT('Ctrl Pts',(-90.,-11.4131225018002,-0.687027337826157));
#34942=CARTESIAN_POINT('Ctrl Pts',(-90.,-11.4195212522844,-0.621218378851216));
#34943=CARTESIAN_POINT('Ctrl Pts',(-90.,-11.4253563443557,-0.555329287367791));
#34944=CARTESIAN_POINT('Ctrl Pts',(-90.,-11.4306253562291,-0.489367343649453));
#34945=CARTESIAN_POINT('Ctrl Pts',(-90.,-11.4328878359414,-0.461043710484138));
#34946=CARTESIAN_POINT('Ctrl Pts',(-90.,-11.4350458220249,-0.432707732928388));
#34947=CARTESIAN_POINT('Ctrl Pts',(-90.,-11.4370983178205,-0.404372587164961));
#34948=CARTESIAN_POINT('Ctrl Pts',(-90.,-11.4570807825108,-0.128510365709557));
#34949=CARTESIAN_POINT('Ctrl Pts',(-90.,-11.4670944941131,0.147589620248241));
#34950=CARTESIAN_POINT('Ctrl Pts',(-90.,-11.4671365005577,0.423375648430594));
#34951=CARTESIAN_POINT('Ctrl Pts',(-90.,-11.4671787076057,0.700478703366769));
#34952=CARTESIAN_POINT('Ctrl Pts',(-90.,-11.4571538896401,0.977265418803752));
#34953=CARTESIAN_POINT('Ctrl Pts',(-90.,-11.4370088281763,1.25319083488204));
#34954=CARTESIAN_POINT('Ctrl Pts',(-90.,-11.432234510889,1.31858430545373));
#34955=CARTESIAN_POINT('Ctrl Pts',(-90.,-11.4268915378888,1.38392943996235));
#34956=CARTESIAN_POINT('Ctrl Pts',(-90.,-11.4209787755945,1.44921904475968));
#34957=CARTESIAN_POINT('Ctrl Pts',(-90.,-11.3961509419423,1.72337169396549));
#34958=CARTESIAN_POINT('Ctrl Pts',(-90.,-11.3612808807937,1.99654535611728));
#34959=CARTESIAN_POINT('Ctrl Pts',(-90.,-11.3166035627522,2.26824946846252));
#34960=CARTESIAN_POINT('Ctrl Pts',(-90.,-11.271735562689,2.54111320926694));
#34961=CARTESIAN_POINT('Ctrl Pts',(-90.,-11.2169762691305,2.81249543474008));
#34962=CARTESIAN_POINT('Ctrl Pts',(-90.,-11.1525113673841,3.0818928412696));
#34963=CARTESIAN_POINT('Ctrl Pts',(-90.,-11.1122274203988,3.25023856969861));
#34964=CARTESIAN_POINT('Ctrl Pts',(-90.,-11.0681524360867,3.41780907298995));
#34965=CARTESIAN_POINT('Ctrl Pts',(-90.,-11.0203218032741,3.58447865336719));
#34966=CARTESIAN_POINT('Ctrl Pts',(-90.,-10.9993959014186,3.65739659478223));
#34967=CARTESIAN_POINT('Ctrl Pts',(-90.,-10.9777510486049,3.73014205804691));
#34968=CARTESIAN_POINT('Ctrl Pts',(-90.,-10.9553897639952,3.80270433013029));
#34969=CARTESIAN_POINT('Ctrl Pts',(-90.,-10.9412121665118,3.84871057279642));
#34970=CARTESIAN_POINT('Ctrl Pts',(-90.,-10.9267465675327,3.89464317259038));
#34971=CARTESIAN_POINT('Ctrl Pts',(-90.,-10.9119935538308,3.94049937157543));
#34972=CARTESIAN_POINT('Ctrl Pts',(-90.,-10.9032483052371,3.96768187596365));
#34973=CARTESIAN_POINT('Ctrl Pts',(-90.,-10.89440279516,3.99483517031346));
#34974=CARTESIAN_POINT('Ctrl Pts',(-90.,-10.8854606880556,4.02194834272));
#34975=CARTESIAN_POINT('Ctrl Pts',(-90.,-10.798021459592,4.2870709641265));
#34976=CARTESIAN_POINT('Ctrl Pts',(-90.,-10.7012600918437,4.54863915252615));
#34977=CARTESIAN_POINT('Ctrl Pts',(-90.,-10.5954597983809,4.80616392461528));
#34978=CARTESIAN_POINT('Ctrl Pts',(-90.,-10.4890736553727,5.06511469247184));
#34979=CARTESIAN_POINT('Ctrl Pts',(-90.,-10.373548046733,5.31997775056167));
#34980=CARTESIAN_POINT('Ctrl Pts',(-90.,-10.2491181879724,5.57025027534674));
#34981=CARTESIAN_POINT('Ctrl Pts',(-90.,-10.1249181352476,5.82006057878593));
#34982=CARTESIAN_POINT('Ctrl Pts',(-90.,-9.99184647791854,6.06529789265079));
#34983=CARTESIAN_POINT('Ctrl Pts',(-90.,-9.85008764641507,6.30544744759558));
#34984=CARTESIAN_POINT('Ctrl Pts',(-90.,-9.7374400125352,6.49628056081274));
#34985=CARTESIAN_POINT('Ctrl Pts',(-90.,-9.61930580768373,6.6839008000223));
#34986=CARTESIAN_POINT('Ctrl Pts',(-90.,-9.49575654832475,6.86803937657834));
#34987=CARTESIAN_POINT('Ctrl Pts',(-90.,-9.35867483321646,7.07234680847123));
#34988=CARTESIAN_POINT('Ctrl Pts',(-90.,-9.21492707314738,7.27236859511388));
#34989=CARTESIAN_POINT('Ctrl Pts',(-90.,-9.06478201620882,7.46786749211994));
#34990=CARTESIAN_POINT('Ctrl Pts',(-90.,-8.9990935537982,7.5533982595601));
#34991=CARTESIAN_POINT('Ctrl Pts',(-90.,-8.93218029389725,7.63806306074812));
#34992=CARTESIAN_POINT('Ctrl Pts',(-90.,-8.86406334867798,7.72184075141948));
#34993=CARTESIAN_POINT('Ctrl Pts',(-90.,-8.82362294761177,7.77157879237602));
#34994=CARTESIAN_POINT('Ctrl Pts',(-90.,-8.78275826967116,7.82100413914672));
#34995=CARTESIAN_POINT('Ctrl Pts',(-90.,-8.74147360307109,7.8701122254124));
#34996=CARTESIAN_POINT('Ctrl Pts',(-90.,-8.7177941394386,7.89827893326192));
#34997=CARTESIAN_POINT('Ctrl Pts',(-90.,-8.69397447251461,7.92634356643258));
#34998=CARTESIAN_POINT('Ctrl Pts',(-90.,-8.67003176357098,7.95428637439746));
#34999=CARTESIAN_POINT('Ctrl Pts',(-90.,-8.48862974410169,8.16599515832848));
#35000=CARTESIAN_POINT('Ctrl Pts',(-90.,-8.2999844948834,8.37093434225391));
#35001=CARTESIAN_POINT('Ctrl Pts',(-90.,-8.10458119986093,8.56883289310171));
#35002=CARTESIAN_POINT('Ctrl Pts',(-90.,-7.90691879422699,8.76901940289187));
#35003=CARTESIAN_POINT('Ctrl Pts',(-90.,-7.70234081506854,8.96200199713272));
#35004=CARTESIAN_POINT('Ctrl Pts',(-90.,-7.49130282760398,9.14747446805371));
#35005=CARTESIAN_POINT('Ctrl Pts',(-90.,-7.27896365425757,9.3340904968883));
#35006=CARTESIAN_POINT('Ctrl Pts',(-90.,-7.06008414942282,9.51310396944825));
#35007=CARTESIAN_POINT('Ctrl Pts',(-90.,-6.83508736441859,9.68417023041306));
#35008=CARTESIAN_POINT('Ctrl Pts',(-90.,-6.61081877650966,9.85468283922532));
#35009=CARTESIAN_POINT('Ctrl Pts',(-90.,-6.38047196958125,10.0173000112399));
#35010=CARTESIAN_POINT('Ctrl Pts',(-90.,-6.14443205975055,10.1716414832551));
#35011=CARTESIAN_POINT('Ctrl Pts',(-90.,-5.91150572303173,10.323947056097));
#35012=CARTESIAN_POINT('Ctrl Pts',(-90.,-5.67303499954604,10.468194147758));
#35013=CARTESIAN_POINT('Ctrl Pts',(-90.,-5.42936414325409,10.6039739276061));
#35014=CARTESIAN_POINT('Ctrl Pts',(-90.,-5.33030982339919,10.6591695876353));
#35015=CARTESIAN_POINT('Ctrl Pts',(-90.,-5.23039592609036,10.7129654986999));
#35016=CARTESIAN_POINT('Ctrl Pts',(-90.,-5.12964461189318,10.765331911078));
#35017=CARTESIAN_POINT('Origin',(-92.9267766952966,0.,-4.79034268955998E-16));
#35018=CARTESIAN_POINT('',(-93.3535533905933,15.6464466094067,1.91613707582399E-15));
#35019=CARTESIAN_POINT('',(-92.9267766952966,15.8232233047034,1.93778597722988E-15));
#35020=CARTESIAN_POINT('',(-93.3535533905933,-15.6464466094067,-1.91613707582399E-15));
#35021=CARTESIAN_POINT('Origin',(-93.3535533905933,0.,-9.58068537911996E-16));
#35022=CARTESIAN_POINT('Origin',(-93.3535533905933,0.,-9.58068537911996E-16));
#35023=CARTESIAN_POINT('Origin',(-93.5,0.,0.));
#35024=CARTESIAN_POINT('',(-93.6464466094067,-15.3535533905933,-1.88026800153281E-15));
#35025=CARTESIAN_POINT('',(-93.5,-15.5,-1.8982025386784E-15));
#35026=CARTESIAN_POINT('',(-93.6464466094067,15.3535533905933,-1.88026800153281E-15));
#35027=CARTESIAN_POINT('Origin',(-93.6464466094067,0.,-9.40134000766403E-16));
#35028=CARTESIAN_POINT('Origin',(-93.6464466094067,0.,-9.40134000766403E-16));
#35029=CARTESIAN_POINT('Origin',(-93.8232233047034,0.,-4.70067000383201E-16));
#35030=CARTESIAN_POINT('',(-94.,14.5,1.77573785876366E-15));
#35031=CARTESIAN_POINT('',(-93.8232233047034,14.9267766952966,1.82800293014823E-15));
#35032=CARTESIAN_POINT('Origin',(-94.,0.,0.));
#35033=CARTESIAN_POINT('Origin',(-94.,15.,0.));
#35034=CARTESIAN_POINT('',(-94.,5.5,-3.17542648054294));
#35035=CARTESIAN_POINT('',(-94.,-3.88578058618805E-15,-6.35085296108589));
#35036=CARTESIAN_POINT('',(-94.,7.125,-2.2372322931098));
#35037=CARTESIAN_POINT('',(-94.,5.5,3.17542648054294));
#35038=CARTESIAN_POINT('',(-94.,5.5,-1.44337567297406));
#35039=CARTESIAN_POINT('',(-94.,-6.66133814775094E-15,6.35085296108589));
#35040=CARTESIAN_POINT('',(-94.,9.625,0.793856620135735));
#35041=CARTESIAN_POINT('',(-94.,-5.50000000000001,3.17542648054294));
#35042=CARTESIAN_POINT('',(-94.,4.125,8.73242282149309));
#35043=CARTESIAN_POINT('',(-94.,-5.5,-3.17542648054295));
#35044=CARTESIAN_POINT('',(-94.,-5.5,1.44337567297406));
#35045=CARTESIAN_POINT('',(-94.,1.625,-7.28904714851903));
#35046=CARTESIAN_POINT('Origin',(-93.75,4.25,8.51591647054698));
#35047=CARTESIAN_POINT('',(-93.5,3.53525079574969E-16,5.77350269189626));
#35048=CARTESIAN_POINT('',(-94.,-4.44089209850063E-15,6.35085296108589));
#35049=CARTESIAN_POINT('',(-93.5,-5.,2.88675134594813));
#35050=CARTESIAN_POINT('',(-93.5,4.375,8.29941011960087));
#35051=CARTESIAN_POINT('',(-94.,-5.5,3.17542648054295));
#35052=CARTESIAN_POINT('Origin',(-93.75,9.5,0.577350269189625));
#35053=CARTESIAN_POINT('',(-93.5,5.,2.88675134594813));
#35054=CARTESIAN_POINT('',(-94.,5.5,3.17542648054294));
#35055=CARTESIAN_POINT('',(-93.5,9.375,0.360843918243515));
#35056=CARTESIAN_POINT('Origin',(-93.75,7.,-2.02072594216369));
#35057=CARTESIAN_POINT('',(-93.5,-1.06057523872491E-15,-5.77350269189626));
#35058=CARTESIAN_POINT('',(-94.,-3.88578058618805E-15,-6.35085296108589));
#35059=CARTESIAN_POINT('',(-93.5,5.,-2.88675134594813));
#35060=CARTESIAN_POINT('',(-93.5,6.875,-1.80421959121758));
#35061=CARTESIAN_POINT('',(-93.5,5.,-2.88675134594813));
#35062=CARTESIAN_POINT('Origin',(-93.75,1.75,-7.07254079757292));
#35063=CARTESIAN_POINT('',(-93.5,-5.,-2.88675134594813));
#35064=CARTESIAN_POINT('',(-93.5,1.875,-6.85603444662681));
#35065=CARTESIAN_POINT('',(-94.,-5.5,-3.17542648054295));
#35066=CARTESIAN_POINT('Origin',(-93.75,5.25,-1.44337567297406));
#35067=CARTESIAN_POINT('',(-93.5,5.,-1.44337567297406));
#35068=CARTESIAN_POINT('Origin',(-93.75,-5.25,1.44337567297406));
#35069=CARTESIAN_POINT('',(-93.5,-5.,1.44337567297406));
#35070=CARTESIAN_POINT('Origin',(-94.,5.,2.88675134594813));
#35071=CARTESIAN_POINT('',(-89.,5.,2.88675134594813));
#35072=CARTESIAN_POINT('',(-94.,5.,2.88675134594813));
#35073=CARTESIAN_POINT('',(-89.,5.55111512312578E-16,5.77350269189626));
#35074=CARTESIAN_POINT('',(-89.,5.,2.88675134594813));
#35075=CARTESIAN_POINT('',(-94.,3.53525079574969E-16,5.77350269189626));
#35076=CARTESIAN_POINT('Origin',(-94.,5.,-2.88675134594813));
#35077=CARTESIAN_POINT('',(-89.,5.,-2.88675134594813));
#35078=CARTESIAN_POINT('',(-94.,5.,-2.88675134594813));
#35079=CARTESIAN_POINT('',(-89.,5.,-2.88675134594813));
#35080=CARTESIAN_POINT('Origin',(-94.,-1.06057523872491E-15,-5.77350269189626));
#35081=CARTESIAN_POINT('',(-89.,-1.11022302462516E-15,-5.77350269189626));
#35082=CARTESIAN_POINT('',(-94.,-1.06057523872491E-15,-5.77350269189626));
#35083=CARTESIAN_POINT('',(-89.,-1.06057523872491E-15,-5.77350269189626));
#35084=CARTESIAN_POINT('Origin',(-81.425,1.39622887047493E-15,0.));
#35085=CARTESIAN_POINT('',(-81.425,9.46357049537274,-7.25578792958495));
#35086=CARTESIAN_POINT('Ctrl Pts',(-81.425,-10.1493211523489,-4.41097929944942));
#35087=CARTESIAN_POINT('Ctrl Pts',(-81.425,-10.0511972777313,-4.66274678383263));
#35088=CARTESIAN_POINT('Ctrl Pts',(-81.425,-9.94393250654178,-4.91057796500162));
#35089=CARTESIAN_POINT('Ctrl Pts',(-81.425,-9.82767522759895,-5.15394628116773));
#35090=CARTESIAN_POINT('Ctrl Pts',(-81.425,-9.82022016054204,-5.16955241897728));
#35091=CARTESIAN_POINT('Ctrl Pts',(-81.425,-9.81272809794668,-5.18514020202351));
#35092=CARTESIAN_POINT('Ctrl Pts',(-81.425,-9.80519907176881,-5.20070949003747));
#35093=CARTESIAN_POINT('Ctrl Pts',(-81.425,-9.68859202725284,-5.44184142631154));
#35094=CARTESIAN_POINT('Ctrl Pts',(-81.425,-9.56312278215398,-5.67853847881199));
#35095=CARTESIAN_POINT('Ctrl Pts',(-81.425,-9.42919331651251,-5.91043494040433));
#35096=CARTESIAN_POINT('Ctrl Pts',(-81.425,-9.29444350025844,-6.1437518243318));
#35097=CARTESIAN_POINT('Ctrl Pts',(-81.425,-9.15112916840663,-6.37220964860501));
#35098=CARTESIAN_POINT('Ctrl Pts',(-81.425,-8.99961185123732,-6.59541327943604));
#35099=CARTESIAN_POINT('Ctrl Pts',(-81.425,-8.95289617696045,-6.66423120936062));
#35100=CARTESIAN_POINT('Ctrl Pts',(-81.425,-8.90540040001368,-6.73254947992113));
#35101=CARTESIAN_POINT('Ctrl Pts',(-81.425,-8.85713428342694,-6.8003559591904));
#35102=CARTESIAN_POINT('Ctrl Pts',(-81.425,-8.82981577402108,-6.83873426829606));
#35103=CARTESIAN_POINT('Ctrl Pts',(-81.425,-8.80225047688398,-6.87694861825185));
#35104=CARTESIAN_POINT('Ctrl Pts',(-81.425,-8.774440110005,-6.91499676774056));
#35105=CARTESIAN_POINT('Ctrl Pts',(-81.425,-8.75328251436771,-6.94394307273295));
#35106=CARTESIAN_POINT('Ctrl Pts',(-81.425,-8.73198276368499,-6.97279352399088));
#35107=CARTESIAN_POINT('Ctrl Pts',(-81.425,-8.71055099837558,-7.00153474506046));
#35108=CARTESIAN_POINT('Ctrl Pts',(-81.425,-8.5488453047104,-7.21839131393111));
#35109=CARTESIAN_POINT('Ctrl Pts',(-81.425,-8.37950258163264,-7.4292042102773));
#35110=CARTESIAN_POINT('Ctrl Pts',(-81.425,-8.2029322943441,-7.63360703972012));
#35111=CARTESIAN_POINT('Ctrl Pts',(-81.425,-8.02514413249846,-7.83941971568467));
#35112=CARTESIAN_POINT('Ctrl Pts',(-81.425,-7.84002801022476,-8.03873412469252));
#35113=CARTESIAN_POINT('Ctrl Pts',(-81.425,-7.64795639954535,-8.23115004848213));
#35114=CARTESIAN_POINT('Ctrl Pts',(-81.425,-7.45646368826431,-8.42298603512162));
#35115=CARTESIAN_POINT('Ctrl Pts',(-81.425,-7.2580569377017,-8.60796554982375));
#35116=CARTESIAN_POINT('Ctrl Pts',(-81.425,-7.05306601649295,-8.78565843431322));
#35117=CARTESIAN_POINT('Ctrl Pts',(-81.425,-6.98673167123628,-8.84315923034786));
#35118=CARTESIAN_POINT('Ctrl Pts',(-81.425,-6.91970758521381,-8.89989671529736));
#35119=CARTESIAN_POINT('Ctrl Pts',(-81.425,-6.85200416263363,-8.95585542472905));
#35120=CARTESIAN_POINT('Ctrl Pts',(-81.425,-6.81464616008689,-8.98673282397701));
#35121=CARTESIAN_POINT('Ctrl Pts',(-81.425,-6.77708131288144,-9.01737310047241));
#35122=CARTESIAN_POINT('Ctrl Pts',(-81.425,-6.73931132370747,-9.04777359412434));
#35123=CARTESIAN_POINT('Ctrl Pts',(-81.425,-6.71515665375601,-9.06721532303619));
#35124=CARTESIAN_POINT('Ctrl Pts',(-81.425,-6.69092198364463,-9.08655581632656));
#35125=CARTESIAN_POINT('Ctrl Pts',(-81.425,-6.66661386320815,-9.1057897743195));
#35126=CARTESIAN_POINT('Ctrl Pts',(-81.425,-6.52227718275629,-9.21999710910322));
#35127=CARTESIAN_POINT('Ctrl Pts',(-81.425,-6.37528765951429,-9.33050025169547));
#35128=CARTESIAN_POINT('Ctrl Pts',(-81.425,-6.22576844769021,-9.43718820340569));
#35129=CARTESIAN_POINT('Ctrl Pts',(-81.425,-6.00610153703119,-9.59392935038481));
#35130=CARTESIAN_POINT('Ctrl Pts',(-81.425,-5.78097625235967,-9.74243767872015));
#35131=CARTESIAN_POINT('Ctrl Pts',(-81.425,-5.55093786621179,-9.88262226273903));
#35132=CARTESIAN_POINT('Ctrl Pts',(-81.425,-5.31834583144998,-10.0243630312481));
#35133=CARTESIAN_POINT('Ctrl Pts',(-81.425,-5.0807305129784,-10.1575945320724));
#35134=CARTESIAN_POINT('Ctrl Pts',(-81.425,-4.83861901722481,-10.2821832996586));
#35135=CARTESIAN_POINT('Ctrl Pts',(-81.425,-4.59524814941176,-10.4074201307014));
#35136=CARTESIAN_POINT('Ctrl Pts',(-81.425,-4.34733365355969,-10.5239243712292));
#35137=CARTESIAN_POINT('Ctrl Pts',(-81.425,-4.09538219844386,-10.6315163530296));
#35138=CARTESIAN_POINT('Ctrl Pts',(-81.425,-3.84587529675822,-10.7380644260021));
#35139=CARTESIAN_POINT('Ctrl Pts',(-81.425,-3.59240879618425,-10.8358725233087));
#35140=CARTESIAN_POINT('Ctrl Pts',(-81.425,-3.33545536944063,-10.9247196817515));
#35141=CARTESIAN_POINT('Ctrl Pts',(-81.425,-3.23909783441178,-10.9580373661676));
#35142=CARTESIAN_POINT('Ctrl Pts',(-81.425,-3.14224979922048,-10.9900944331567));
#35143=CARTESIAN_POINT('Ctrl Pts',(-81.425,-3.0449357380293,-11.0208774396873));
#35144=CARTESIAN_POINT('Ctrl Pts',(-81.425,-2.98189523387823,-11.0408188153449));
#35145=CARTESIAN_POINT('Ctrl Pts',(-81.425,-2.91865915728009,-11.0602255101925));
#35146=CARTESIAN_POINT('Ctrl Pts',(-81.425,-2.85523412591873,-11.0790936417007));
#35147=CARTESIAN_POINT('Ctrl Pts',(-81.425,-2.82799982747709,-11.0871954953932));
#35148=CARTESIAN_POINT('Ctrl Pts',(-81.425,-2.80073172898171,-11.0951977054104));
#35149=CARTESIAN_POINT('Ctrl Pts',(-81.425,-2.77344251147326,-11.1030965573882));
#35150=CARTESIAN_POINT('Ctrl Pts',(-81.425,-2.50776312916618,-11.1799973374758));
#35151=CARTESIAN_POINT('Ctrl Pts',(-81.425,-2.23977856115638,-11.2471966373664));
#35152=CARTESIAN_POINT('Ctrl Pts',(-81.425,-1.97002786073214,-11.3045768591928));
#35153=CARTESIAN_POINT('Ctrl Pts',(-81.425,-1.69898895910337,-11.3622311017012));
#35154=CARTESIAN_POINT('Ctrl Pts',(-81.425,-1.42616643671568,-11.4099725343039));
#35155=CARTESIAN_POINT('Ctrl Pts',(-81.425,-1.1520822812381,-11.4476357971411));
#35156=CARTESIAN_POINT('Ctrl Pts',(-81.425,-1.08712517140243,-11.4565618756903));
#35157=CARTESIAN_POINT('Ctrl Pts',(-81.425,-1.02209711150722,-11.464921674965));
#35158=CARTESIAN_POINT('Ctrl Pts',(-81.425,-0.957004902337799,-11.4727125904994));
#35159=CARTESIAN_POINT('Ctrl Pts',(-81.425,-0.683681187122471,-11.5054268278247));
#35160=CARTESIAN_POINT('Ctrl Pts',(-81.425,-0.409227175555571,-11.528114738695));
#35161=CARTESIAN_POINT('Ctrl Pts',(-81.425,-0.134171561186469,-11.5409041668509));
#35162=CARTESIAN_POINT('Ctrl Pts',(-81.425,0.14205800605394,-11.5537481810073));
#35163=CARTESIAN_POINT('Ctrl Pts',(-81.425,0.418894944292535,-11.5566090229993));
#35164=CARTESIAN_POINT('Ctrl Pts',(-81.425,0.695808344418892,-11.5495636793336));
#35165=CARTESIAN_POINT('Ctrl Pts',(-81.425,0.868850798209164,-11.5451610626486));
#35166=CARTESIAN_POINT('Ctrl Pts',(-81.425,1.04192316773346,-11.5368890730119));
#35167=CARTESIAN_POINT('Ctrl Pts',(-81.425,1.21489514481341,-11.5247561922664));
#35168=CARTESIAN_POINT('Ctrl Pts',(-81.425,1.29057038478588,-11.5194480569403));
#35169=CARTESIAN_POINT('Ctrl Pts',(-81.425,1.36622639396203,-11.5134008212102));
#35170=CARTESIAN_POINT('Ctrl Pts',(-81.425,1.44185216969932,-11.5066147218566));
#35171=CARTESIAN_POINT('Ctrl Pts',(-81.425,1.48980074839904,-11.5023121700381));
#35172=CARTESIAN_POINT('Ctrl Pts',(-81.425,1.53773717238975,-11.4977125990324));
#35173=CARTESIAN_POINT('Ctrl Pts',(-81.425,1.58565862201697,-11.492816009391));
#35174=CARTESIAN_POINT('Ctrl Pts',(-81.425,1.61406535643,-11.4899134235436));
#35175=CARTESIAN_POINT('Ctrl Pts',(-81.425,1.64246436467114,-11.4869066940838));
#35176=CARTESIAN_POINT('Ctrl Pts',(-81.425,1.67084421139455,-11.4837971366815));
#35177=CARTESIAN_POINT('Ctrl Pts',(-81.425,1.94835285038083,-11.4533907341748));
#35178=CARTESIAN_POINT('Ctrl Pts',(-81.425,2.22432291238045,-11.4131268975024));
#35179=CARTESIAN_POINT('Ctrl Pts',(-81.425,2.49821721852931,-11.363180987543));
#35180=CARTESIAN_POINT('Ctrl Pts',(-81.425,2.77362818031292,-11.3129585083229));
#35181=CARTESIAN_POINT('Ctrl Pts',(-81.425,3.04694096391893,-11.2529464026702));
#35182=CARTESIAN_POINT('Ctrl Pts',(-81.425,3.31761483196776,-11.1832702047752));
#35183=CARTESIAN_POINT('Ctrl Pts',(-81.425,3.58778884299265,-11.1137226788394));
#35184=CARTESIAN_POINT('Ctrl Pts',(-81.425,3.8553343105734,-11.0345466372617));
#35185=CARTESIAN_POINT('Ctrl Pts',(-81.425,4.11970937111498,-10.945815455283));
#35186=CARTESIAN_POINT('Ctrl Pts',(-81.425,4.32979306970644,-10.8753058737351));
#35187=CARTESIAN_POINT('Ctrl Pts',(-81.425,4.53787483073322,-10.7987616258001));
#35188=CARTESIAN_POINT('Ctrl Pts',(-81.425,4.74367687130894,-10.71619678164));
#35189=CARTESIAN_POINT('Ctrl Pts',(-81.425,4.97202059158535,-10.6245885370044));
#35190=CARTESIAN_POINT('Ctrl Pts',(-81.425,5.1975582746143,-10.52556888611));
#35191=CARTESIAN_POINT('Ctrl Pts',(-81.425,5.42000198252274,-10.4193513770082));
#35192=CARTESIAN_POINT('Ctrl Pts',(-81.425,5.51732110473269,-10.3728812167762));
#35193=CARTESIAN_POINT('Ctrl Pts',(-81.425,5.61404783494252,-10.3250329800772));
#35194=CARTESIAN_POINT('Ctrl Pts',(-81.425,5.71015710130799,-10.2758229214779));
#35195=CARTESIAN_POINT('Ctrl Pts',(-81.425,5.76721628348422,-10.2466073650107));
#35196=CARTESIAN_POINT('Ctrl Pts',(-81.425,5.82405781705297,-10.2169117906126));
#35197=CARTESIAN_POINT('Ctrl Pts',(-81.425,5.88067634387593,-10.1867394433756));
#35198=CARTESIAN_POINT('Ctrl Pts',(-81.425,5.91315078310045,-10.1694336229738));
#35199=CARTESIAN_POINT('Ctrl Pts',(-81.425,5.94555452822165,-10.1519694406033));
#35200=CARTESIAN_POINT('Ctrl Pts',(-81.425,5.97786469226987,-10.1343595761495));
#35201=CARTESIAN_POINT('Ctrl Pts',(-81.425,6.22266283943227,-10.0009383349686));
#35202=CARTESIAN_POINT('Ctrl Pts',(-81.425,6.46234527253621,-9.85902466517761));
#35203=CARTESIAN_POINT('Ctrl Pts',(-81.425,6.69654600256747,-9.70903679572445));
#35204=CARTESIAN_POINT('Ctrl Pts',(-81.425,6.93345436614612,-9.55731489159525));
#35205=CARTESIAN_POINT('Ctrl Pts',(-81.425,7.16475406529005,-9.39733075575456));
#35206=CARTESIAN_POINT('Ctrl Pts',(-81.425,7.39005086306915,-9.22946633224029));
#35207=CARTESIAN_POINT('Ctrl Pts',(-81.425,7.61673670522224,-9.0605669577841));
#35208=CARTESIAN_POINT('Ctrl Pts',(-81.425,7.83734593604377,-8.88368951375276));
#35209=CARTESIAN_POINT('Ctrl Pts',(-81.425,8.05145347150729,-8.69917614679468));
#35210=CARTESIAN_POINT('Ctrl Pts',(-81.425,8.26486801649614,-8.51525998443976));
#35211=CARTESIAN_POINT('Ctrl Pts',(-81.425,8.47182339046597,-8.32375687389967));
#35212=CARTESIAN_POINT('Ctrl Pts',(-81.425,8.67186756704869,-8.12496445217349));
#35213=CARTESIAN_POINT('Ctrl Pts',(-81.425,8.86927294001326,-7.92879432203648));
#35214=CARTESIAN_POINT('Ctrl Pts',(-81.425,9.05994867105627,-7.72552551270578));
#35215=CARTESIAN_POINT('Ctrl Pts',(-81.425,9.24342328678313,-7.51540975236948));
#35216=CARTESIAN_POINT('Ctrl Pts',(-81.425,9.31800737273546,-7.42999580087118));
#35217=CARTESIAN_POINT('Ctrl Pts',(-81.425,9.39140101136385,-7.34345002965296));
#35218=CARTESIAN_POINT('Ctrl Pts',(-81.425,9.46357049537284,-7.25578792958482));
#35219=CARTESIAN_POINT('',(-81.425,-11.925,-1.46039130798322E-15));
#35220=CARTESIAN_POINT('Origin',(-81.425,0.,0.));
#35221=CARTESIAN_POINT('',(-81.425,11.5970184578307,2.77968392481168));
#35222=CARTESIAN_POINT('Origin',(-81.425,0.,0.));
#35223=CARTESIAN_POINT('Ctrl Pts',(-81.425,11.5970184578306,2.77968392481176));
#35224=CARTESIAN_POINT('Ctrl Pts',(-81.425,11.5217985042993,3.05261604105638));
#35225=CARTESIAN_POINT('Ctrl Pts',(-81.425,11.4369053700675,3.3225041885107));
#35226=CARTESIAN_POINT('Ctrl Pts',(-81.425,11.3423804739584,3.58881439697669));
#35227=CARTESIAN_POINT('Ctrl Pts',(-81.425,11.3337495693404,3.61313072106369));
#35228=CARTESIAN_POINT('Ctrl Pts',(-81.425,11.3250383282922,3.63741720505413));
#35229=CARTESIAN_POINT('Ctrl Pts',(-81.425,11.3162467616178,3.66167343587083));
#35230=CARTESIAN_POINT('Ctrl Pts',(-81.425,11.2197848936528,3.92781500324165));
#35231=CARTESIAN_POINT('Ctrl Pts',(-81.425,11.113656826452,4.19031635327416));
#35232=CARTESIAN_POINT('Ctrl Pts',(-81.425,10.9981939856909,4.44873106452655));
#35233=CARTESIAN_POINT('Ctrl Pts',(-81.425,10.882655142131,4.70731587588362));
#35234=CARTESIAN_POINT('Ctrl Pts',(-81.425,10.7577688595731,4.9618091896813));
#35235=CARTESIAN_POINT('Ctrl Pts',(-81.425,10.6238227842739,5.21173643838379));
#35236=CARTESIAN_POINT('Ctrl Pts',(-81.425,10.5801769878256,5.29317423937485));
#35237=CARTESIAN_POINT('Ctrl Pts',(-81.425,10.5355689345581,5.37412698664962));
#35238=CARTESIAN_POINT('Ctrl Pts',(-81.425,10.490007659337,5.45457749292015));
#35239=CARTESIAN_POINT('Ctrl Pts',(-81.425,10.4587925795726,5.50969598901436));
#35240=CARTESIAN_POINT('Ctrl Pts',(-81.425,10.4271300544444,5.56457872818468));
#35241=CARTESIAN_POINT('Ctrl Pts',(-81.425,10.3950228757915,5.61922006877392));
#35242=CARTESIAN_POINT('Ctrl Pts',(-81.425,10.3758763329037,5.65180445690571));
#35243=CARTESIAN_POINT('Ctrl Pts',(-81.425,10.3565762277333,5.68429520631596));
#35244=CARTESIAN_POINT('Ctrl Pts',(-81.425,10.3371255444104,5.71668767315294));
#35245=CARTESIAN_POINT('Ctrl Pts',(-81.425,10.1920782333509,5.95824423624583));
#35246=CARTESIAN_POINT('Ctrl Pts',(-81.425,10.0386228839365,6.19440246598055));
#35247=CARTESIAN_POINT('Ctrl Pts',(-81.425,9.87708819968873,6.42472561727724));
#35248=CARTESIAN_POINT('Ctrl Pts',(-81.425,9.71585158140852,6.65462377320365));
#35249=CARTESIAN_POINT('Ctrl Pts',(-81.425,9.54656502423558,6.87870885973711));
#35250=CARTESIAN_POINT('Ctrl Pts',(-81.425,9.36951408979584,7.09651568591001));
#35251=CARTESIAN_POINT('Ctrl Pts',(-81.425,9.19379661890504,7.3126820945142));
#35252=CARTESIAN_POINT('Ctrl Pts',(-81.425,9.01043088264205,7.52266490201881));
#35253=CARTESIAN_POINT('Ctrl Pts',(-81.425,8.81966127669493,7.72597196868344));
#35254=CARTESIAN_POINT('Ctrl Pts',(-81.425,8.75720458209991,7.79253334416378));
#35255=CARTESIAN_POINT('Ctrl Pts',(-81.425,8.69395404007734,7.85837884269289));
#35256=CARTESIAN_POINT('Ctrl Pts',(-81.425,8.62991751890671,7.92349018984214));
#35257=CARTESIAN_POINT('Ctrl Pts',(-81.425,8.59909107785625,7.95483403969408));
#35258=CARTESIAN_POINT('Ctrl Pts',(-81.425,8.56808249318198,7.98600775332298));
#35259=CARTESIAN_POINT('Ctrl Pts',(-81.425,8.5368926161356,8.01700924783947));
#35260=CARTESIAN_POINT('Ctrl Pts',(-81.425,8.51322858239342,8.04053035410114));
#35261=CARTESIAN_POINT('Ctrl Pts',(-81.425,8.48945955094811,8.06395289139918));
#35262=CARTESIAN_POINT('Ctrl Pts',(-81.425,8.46559774965978,8.08726451773069));
#35263=CARTESIAN_POINT('Ctrl Pts',(-81.425,8.32491115744231,8.22470733807765));
#35264=CARTESIAN_POINT('Ctrl Pts',(-81.425,8.18090552595728,8.35839051249524));
#35265=CARTESIAN_POINT('Ctrl Pts',(-81.425,8.03369044282327,8.48816827575853));
#35266=CARTESIAN_POINT('Ctrl Pts',(-81.425,7.82571847091705,8.67150640090755));
#35267=CARTESIAN_POINT('Ctrl Pts',(-81.425,7.61134266473933,8.84705219851411));
#35268=CARTESIAN_POINT('Ctrl Pts',(-81.425,7.39107933880561,9.01461840461428));
#35269=CARTESIAN_POINT('Ctrl Pts',(-81.425,7.16933642874079,9.18331021025947));
#35270=CARTESIAN_POINT('Ctrl Pts',(-81.425,6.94162608609123,9.34391517153392));
#35271=CARTESIAN_POINT('Ctrl Pts',(-81.425,6.70844294298095,9.49620001683205));
#35272=CARTESIAN_POINT('Ctrl Pts',(-81.425,6.47531259544572,9.64845038293982));
#35273=CARTESIAN_POINT('Ctrl Pts',(-81.425,6.23671134404916,9.79238467087765));
#35274=CARTESIAN_POINT('Ctrl Pts',(-81.425,5.99311001119096,9.92772342358337));
#35275=CARTESIAN_POINT('Ctrl Pts',(-81.425,5.7535262708949,10.0608301032546));
#35276=CARTESIAN_POINT('Ctrl Pts',(-81.425,5.50910543535088,10.1856225652663));
#35277=CARTESIAN_POINT('Ctrl Pts',(-81.425,5.26028139661988,10.3017873386497));
#35278=CARTESIAN_POINT('Ctrl Pts',(-81.425,5.16697238209576,10.3453491286685));
#35279=CARTESIAN_POINT('Ctrl Pts',(-81.425,5.07304406823687,10.3876971542603));
#35280=CARTESIAN_POINT('Ctrl Pts',(-81.425,4.97851906691336,10.4288130563816));
#35281=CARTESIAN_POINT('Ctrl Pts',(-81.425,4.91387906031031,10.456929767806));
#35282=CARTESIAN_POINT('Ctrl Pts',(-81.425,4.84896001780061,10.4844702710005));
#35283=CARTESIAN_POINT('Ctrl Pts',(-81.425,4.78376915312182,10.5114284151287));
#35284=CARTESIAN_POINT('Ctrl Pts',(-81.425,4.75705838983725,10.5224740211342));
#35285=CARTESIAN_POINT('Ctrl Pts',(-81.425,4.73030228286874,10.5334217009663));
#35286=CARTESIAN_POINT('Ctrl Pts',(-81.425,4.70351414680798,10.5442659500702));
#35287=CARTESIAN_POINT('Ctrl Pts',(-81.425,4.44714165051129,10.6480494759911));
#35288=CARTESIAN_POINT('Ctrl Pts',(-81.425,4.18753935832216,10.7424874791396));
#35289=CARTESIAN_POINT('Ctrl Pts',(-81.425,3.92519186134608,10.8273725124873));
#35290=CARTESIAN_POINT('Ctrl Pts',(-81.425,3.66337816313301,10.9120848301571));
#35291=CARTESIAN_POINT('Ctrl Pts',(-81.425,3.39882983789161,10.9872832448377));
#35292=CARTESIAN_POINT('Ctrl Pts',(-81.425,3.13200923994814,11.0527136217828));
#35293=CARTESIAN_POINT('Ctrl Pts',(-81.425,3.06437294932055,11.0692995526482));
#35294=CARTESIAN_POINT('Ctrl Pts',(-81.425,2.99659057691665,11.0852575675369));
#35295=CARTESIAN_POINT('Ctrl Pts',(-81.425,2.92866952489536,11.1005830083263));
#35296=CARTESIAN_POINT('Ctrl Pts',(-81.425,2.65985117950432,11.1612381294237));
#35297=CARTESIAN_POINT('Ctrl Pts',(-81.425,2.38886085810285,11.211988549086));
#35298=CARTESIAN_POINT('Ctrl Pts',(-81.425,2.11624750393544,11.2528573135585));
#35299=CARTESIAN_POINT('Ctrl Pts',(-81.425,1.84398138595298,11.293674022203));
#35300=CARTESIAN_POINT('Ctrl Pts',(-81.425,1.57009572128014,11.3246341879216));
#35301=CARTESIAN_POINT('Ctrl Pts',(-81.425,1.29513858687471,11.3457089466435));
#35302=CARTESIAN_POINT('Ctrl Pts',(-81.425,1.12731412368966,11.358572261054));
#35303=CARTESIAN_POINT('Ctrl Pts',(-81.425,0.959090553024955,11.3677517951114));
#35304=CARTESIAN_POINT('Ctrl Pts',(-81.425,0.790594291629415,11.3732315749573));
#35305=CARTESIAN_POINT('Ctrl Pts',(-81.425,0.716877177268866,11.3756289786399));
#35306=CARTESIAN_POINT('Ctrl Pts',(-81.425,0.643107892631068,11.3773181344974));
#35307=CARTESIAN_POINT('Ctrl Pts',(-81.425,0.569297156125015,11.3782972772602));
#35308=CARTESIAN_POINT('Ctrl Pts',(-81.425,0.521054888586819,11.3789372392679));
#35309=CARTESIAN_POINT('Ctrl Pts',(-81.425,0.472794915191581,11.3792738887815));
#35310=CARTESIAN_POINT('Ctrl Pts',(-81.425,0.424520251078811,11.3793066729465));
#35311=CARTESIAN_POINT('Ctrl Pts',(-81.425,0.39874870013549,11.3793241748554));
#35312=CARTESIAN_POINT('Ctrl Pts',(-81.425,0.372975281400623,11.3792550536749));
#35313=CARTESIAN_POINT('Ctrl Pts',(-81.425,0.347209175026665,11.3790993778194));
#35314=CARTESIAN_POINT('Ctrl Pts',(-81.425,0.0734815860316532,11.3774455471641));
#35315=CARTESIAN_POINT('Ctrl Pts',(-81.425,-0.199703083913748,11.3660280134118));
#35316=CARTESIAN_POINT('Ctrl Pts',(-81.425,-0.471811801903946,11.3449168432811));
#35317=CARTESIAN_POINT('Ctrl Pts',(-81.425,-0.744128229367082,11.3237895583046));
#35318=CARTESIAN_POINT('Ctrl Pts',(-81.425,-1.01536770403303,11.2929537790733));
#35319=CARTESIAN_POINT('Ctrl Pts',(-81.425,-1.28499555980274,11.252427519917));
#35320=CARTESIAN_POINT('Ctrl Pts',(-81.425,-1.55216598200515,11.2122706238938));
#35321=CARTESIAN_POINT('Ctrl Pts',(-81.425,-1.81775462924585,11.162598960697));
#35322=CARTESIAN_POINT('Ctrl Pts',(-81.425,-2.08123166878887,11.103380257873));
#35323=CARTESIAN_POINT('Ctrl Pts',(-81.425,-2.28947413933727,11.0565759936376));
#35324=CARTESIAN_POINT('Ctrl Pts',(-81.425,-2.4963974611547,11.0038069733648));
#35325=CARTESIAN_POINT('Ctrl Pts',(-81.425,-2.70173202408833,10.9450356164872));
#35326=CARTESIAN_POINT('Ctrl Pts',(-81.425,-2.92532867485418,10.8810372405146));
#35327=CARTESIAN_POINT('Ctrl Pts',(-81.425,-3.14704176006627,10.809921422957));
#35328=CARTESIAN_POINT('Ctrl Pts',(-81.425,-3.36656764435611,10.7318318227437));
#35329=CARTESIAN_POINT('Ctrl Pts',(-81.425,-3.46261021873292,10.6976676226504));
#35330=CARTESIAN_POINT('Ctrl Pts',(-81.425,-3.55823395247638,10.6621683008846));
#35331=CARTESIAN_POINT('Ctrl Pts',(-81.425,-3.65341241758583,10.6253445554974));
#35332=CARTESIAN_POINT('Ctrl Pts',(-81.425,-3.71475354916237,10.60161218906));
#35333=CARTESIAN_POINT('Ctrl Pts',(-81.425,-3.77590972035012,10.577329692097));
#35334=CARTESIAN_POINT('Ctrl Pts',(-81.425,-3.83687370523298,10.5524997600722));
#35335=CARTESIAN_POINT('Ctrl Pts',(-81.425,-3.87031237457408,10.53888057346));
#35336=CARTESIAN_POINT('Ctrl Pts',(-81.425,-3.90369614804835,10.5250954090512));
#35337=CARTESIAN_POINT('Ctrl Pts',(-81.425,-3.93700061106458,10.511154572755));
#35338=CARTESIAN_POINT('Ctrl Pts',(-81.425,-4.18507021673326,10.4073157040421));
#35339=CARTESIAN_POINT('Ctrl Pts',(-81.425,-4.42899972961956,10.2947407144357));
#35340=CARTESIAN_POINT('Ctrl Pts',(-81.425,-4.66837293118891,10.1737602696767));
#35341=CARTESIAN_POINT('Ctrl Pts',(-81.425,-4.90946801249104,10.0519095780624));
#35342=CARTESIAN_POINT('Ctrl Pts',(-81.425,-5.14594155284255,9.92153176711564));
#35343=CARTESIAN_POINT('Ctrl Pts',(-81.425,-5.37734790134712,9.78291608734042));
#35344=CARTESIAN_POINT('Ctrl Pts',(-81.425,-5.60826968673858,9.64459066773201));
#35345=CARTESIAN_POINT('Ctrl Pts',(-81.425,-5.83414600053385,9.4980614796471));
#35346=CARTESIAN_POINT('Ctrl Pts',(-81.425,-6.05450572023333,9.34357285602055));
#35347=CARTESIAN_POINT('Ctrl Pts',(-81.425,-6.27316081046619,9.19027930498009));
#35348=CARTESIAN_POINT('Ctrl Pts',(-81.425,-6.48638479737507,9.02914860957272));
#35349=CARTESIAN_POINT('Ctrl Pts',(-81.425,-6.69368220069637,8.8603825530767));
#35350=CARTESIAN_POINT('Ctrl Pts',(-81.425,-6.89733986369601,8.69457970118872));
#35351=CARTESIAN_POINT('Ctrl Pts',(-81.425,-7.09527760205493,8.52140687138442));
#35352=CARTESIAN_POINT('Ctrl Pts',(-81.425,-7.28698538174064,8.34102533285908));
#35353=CARTESIAN_POINT('Ctrl Pts',(-81.425,-7.35124004705837,8.28056688194778));
#35354=CARTESIAN_POINT('Ctrl Pts',(-81.425,-7.41479448322397,8.21929838490928));
#35355=CARTESIAN_POINT('Ctrl Pts',(-81.425,-7.47762833958605,8.15722525234652));
#35356=CARTESIAN_POINT('Ctrl Pts',(-90.4959727487473,-4.76011662834209,
9.98982177454039));
#35357=CARTESIAN_POINT('Ctrl Pts',(-90.4561877805511,-6.42492926884305,
9.19654412535156));
#35358=CARTESIAN_POINT('Ctrl Pts',(-90.3766178441586,-9.3484606603926,6.76207805195742));
#35359=CARTESIAN_POINT('Ctrl Pts',(-90.2572629395698,-11.4459302495084,
1.452207172033));
#35360=CARTESIAN_POINT('Ctrl Pts',(-90.137908034981,-10.7411695159004,-4.21217348791161));
#35361=CARTESIAN_POINT('Ctrl Pts',(-90.0185531303922,-7.40726206096264,
-8.84594083473326));
#35362=CARTESIAN_POINT('Ctrl Pts',(-89.8991982258035,-2.26004805937129,
-11.314084834924));
#35363=CARTESIAN_POINT('Ctrl Pts',(-89.7798433212146,3.44036023950592,-11.0127707789974));
#35364=CARTESIAN_POINT('Ctrl Pts',(-89.6604884166259,8.29862462059312,-8.01559288387814));
#35365=CARTESIAN_POINT('Ctrl Pts',(-89.5411335120371,11.1254633134624,-3.0563078705199));
#35366=CARTESIAN_POINT('Ctrl Pts',(-89.4217786074483,11.2289102651267,2.65114154106624));
#35367=CARTESIAN_POINT('Ctrl Pts',(-89.3024237028595,8.5836358520776,7.70961342848463));
#35368=CARTESIAN_POINT('Ctrl Pts',(-89.1830687982707,3.83717874800117,10.8808559114985));
#35369=CARTESIAN_POINT('Ctrl Pts',(-89.063713893682,-1.84857987243133,11.3885779344766));
#35370=CARTESIAN_POINT('Ctrl Pts',(-88.9443589890932,-7.08182533389115,
9.10849653409288));
#35371=CARTESIAN_POINT('Ctrl Pts',(-88.8250040845044,-10.5815145635538,
4.5987506684781));
#35372=CARTESIAN_POINT('Ctrl Pts',(-88.7056491799156,-11.4909602705537,
-1.03672083502261));
#35373=CARTESIAN_POINT('Ctrl Pts',(-88.5862942753268,-9.58753979769892,
-6.41841405704041));
#35374=CARTESIAN_POINT('Ctrl Pts',(-88.4669393707381,-5.33719041442222,
-10.2289469935215));
#35375=CARTESIAN_POINT('Ctrl Pts',(-88.3475844661493,0.219647037160976,
-11.5355413152965));
#35376=CARTESIAN_POINT('Ctrl Pts',(-88.2282295615605,5.72271720750059,-10.0183564501475));
#35377=CARTESIAN_POINT('Ctrl Pts',(-88.1088746569716,9.82492639772949,-6.0487833070047));
#35378=CARTESIAN_POINT('Ctrl Pts',(-87.989519752383,11.5220969489527,-0.598531631862895));
#35379=CARTESIAN_POINT('Ctrl Pts',(-87.8701648477941,10.3987793606657,4.99823429024215));
#35380=CARTESIAN_POINT('Ctrl Pts',(-87.7508099432054,6.72994996350157,9.37148503193342));
#35381=CARTESIAN_POINT('Ctrl Pts',(-87.6314550386166,1.41369960344878,11.4506948105535));
#35382=CARTESIAN_POINT('Ctrl Pts',(-87.5121001340278,-4.24860954964163,
10.7268949425594));
#35383=CARTESIAN_POINT('Ctrl Pts',(-87.3927452294391,-8.87090377354262,
7.37726402227169));
#35384=CARTESIAN_POINT('Ctrl Pts',(-87.2733903248503,-11.3216940613219,
2.2217564663167));
#35385=CARTESIAN_POINT('Ctrl Pts',(-87.1540354202614,-11.0010527289193,
-3.47761370329691));
#35386=CARTESIAN_POINT('Ctrl Pts',(-87.0346805156727,-7.98746940186916,
-8.32570061724489));
#35387=CARTESIAN_POINT('Ctrl Pts',(-86.9153256110839,-3.01863758058317,
-11.1357435930835));
#35388=CARTESIAN_POINT('Ctrl Pts',(-86.7959707064951,2.68912496921423,-11.2198736674593));
#35389=CARTESIAN_POINT('Ctrl Pts',(-86.6766158019064,7.73861801182051,-8.55749668308028));
#35390=CARTESIAN_POINT('Ctrl Pts',(-86.5572608973175,10.8937787629573,-3.80033452179447));
#35391=CARTESIAN_POINT('Ctrl Pts',(-86.4379059927288,11.3822570579663,1.88710955701514));
#35392=CARTESIAN_POINT('Ctrl Pts',(-86.31855108814,9.08447854823605,7.11260906562713));
#35393=CARTESIAN_POINT('Ctrl Pts',(-86.1991961835512,4.56291524401145,10.5970166881896));
#35394=CARTESIAN_POINT('Ctrl Pts',(-86.0798412789624,-1.07560171741225,
11.4873860890675));
#35395=CARTESIAN_POINT('Ctrl Pts',(-85.9604863743737,-6.45082269201481,
9.56576420418091));
#35396=CARTESIAN_POINT('Ctrl Pts',(-85.8411314697848,-10.2469501238992,
5.30254385857626));
#35397=CARTESIAN_POINT('Ctrl Pts',(-85.7217765651961,-11.5347319468995,
-0.258683449368636));
#35398=CARTESIAN_POINT('Ctrl Pts',(-85.6024216606073,-9.99893271614051,
-5.75658776984223));
#35399=CARTESIAN_POINT('Ctrl Pts',(-85.4830667560185,-6.01549992917226,
-9.84533995430987));
#35400=CARTESIAN_POINT('Ctrl Pts',(-85.3637118514298,-0.559536032933944,
-11.5240564751155));
#35401=CARTESIAN_POINT('Ctrl Pts',(-85.2443569468409,5.03339639874698,-10.3818051853656));
#35402=CARTESIAN_POINT('Ctrl Pts',(-85.1250020422522,9.39420633525482,-6.69819718614323));
#35403=CARTESIAN_POINT('Ctrl Pts',(-85.0056471376634,11.4554133728453,-1.37494097002217));
#35404=CARTESIAN_POINT('Ctrl Pts',(-84.8862922330746,10.7124557092996,4.28488633339115));
#35405=CARTESIAN_POINT('Ctrl Pts',(-84.7669373284858,7.34720156593731,8.89581853250784));
#35406=CARTESIAN_POINT('Ctrl Pts',(-84.647582423897,2.18342975997975,11.3291479245805));
#35407=CARTESIAN_POINT('Ctrl Pts',(-84.5282275193083,-3.5148226850366,10.9892210691436));
#35408=CARTESIAN_POINT('Ctrl Pts',(-84.4088726147195,-8.35268350706726,
7.95924848492489));
#35409=CARTESIAN_POINT('Ctrl Pts',(-84.2895177101306,-11.1458952633209,
2.98093559009735));
#35410=CARTESIAN_POINT('Ctrl Pts',(-84.1701628055419,-11.2107090961286,
-2.72707898253186));
#35411=CARTESIAN_POINT('Ctrl Pts',(-84.0508079009531,-8.53125926061665,
-7.76753330473083));
#35412=CARTESIAN_POINT('Ctrl Pts',(-83.9314529963644,-3.76344689371811,
-10.9065771758865));
#35413=CARTESIAN_POINT('Ctrl Pts',(-83.8120980917756,1.92561768833889,-11.3758056740724));
#35414=CARTESIAN_POINT('Ctrl Pts',(-83.6927431871867,7.1433113126398,-9.06035659838774));
#35415=CARTESIAN_POINT('Ctrl Pts',(-83.573388282598,10.6123974680266,-4.52702752791171));
#35416=CARTESIAN_POINT('Ctrl Pts',(-83.4540333780092,11.4836803397467,1.11447026455969));
#35417=CARTESIAN_POINT('Ctrl Pts',(-83.3346784734204,9.54387907255568,6.48315745825352));
#35418=CARTESIAN_POINT('Ctrl Pts',(-83.2153235688317,5.26783655646332,10.2648358994969));
#35419=CARTESIAN_POINT('Ctrl Pts',(-83.0959686642429,-0.297716860125996,
11.5337904801815));
#35420=CARTESIAN_POINT('Ctrl Pts',(-82.9766137596541,-5.79039248565415,
9.9793944722816));
#35421=CARTESIAN_POINT('Ctrl Pts',(-82.8572588550654,-9.86564059407429,
5.98214765639898));
#35422=CARTESIAN_POINT('Ctrl Pts',(-82.7379039504766,-11.5258843665106,
0.520534034169221));
#35423=CARTESIAN_POINT('Ctrl Pts',(-82.6185490458878,-10.3647114037072,
-5.06850088049748));
#35424=CARTESIAN_POINT('Ctrl Pts',(-82.499194141299,-6.66636917491129,-9.416820017226));
#35425=CARTESIAN_POINT('Ctrl Pts',(-82.3798392367102,-1.33616352515641,
-11.4600008190507));
#35426=CARTESIAN_POINT('Ctrl Pts',(-82.2604843321214,4.32110767959995,-10.6978936382306));
#35427=CARTESIAN_POINT('Ctrl Pts',(-82.1411294275327,8.92064463412699,-7.31705529020618));
#35428=CARTESIAN_POINT('Ctrl Pts',(-82.0217745229439,11.3364445890174,-2.14507737917849));
#35429=CARTESIAN_POINT('Ctrl Pts',(-81.9024196183551,10.9773205983354,3.5519900017792));
#35430=CARTESIAN_POINT('Ctrl Pts',(-81.7830647137664,7.93081818705442,8.37957343457652));
#35431=CARTESIAN_POINT('Ctrl Pts',(-81.6637098091775,2.94344912458979,11.155910191377));
#35432=CARTESIAN_POINT('Ctrl Pts',(-81.5443549045888,-2.76549453716151,
11.2014042094999));
#35433=CARTESIAN_POINT('Ctrl Pts',(-81.4647849681962,-6.11821953149998,
9.40337863342461));
#35434=CARTESIAN_POINT('Ctrl Pts',(-81.425,-7.47762833958605,8.15722525234652));
#35435=CARTESIAN_POINT('Ctrl Pts',(-90.3306484991649,-4.88329262285912,
10.2483251533863));
#35436=CARTESIAN_POINT('Ctrl Pts',(-90.2908635309686,-6.59118508024046,
9.43452011569079));
#35437=CARTESIAN_POINT('Ctrl Pts',(-90.2112935945761,-9.59036774564993,
6.93705815309451));
#35438=CARTESIAN_POINT('Ctrl Pts',(-90.0919386899873,-11.7421128752158,
1.48978546614346));
#35439=CARTESIAN_POINT('Ctrl Pts',(-89.9725837853986,-11.0191152766239,
-4.32117053545506));
#35440=CARTESIAN_POINT('Ctrl Pts',(-89.8532288808097,-7.59893737949893,
-9.07484437740477));
#35441=CARTESIAN_POINT('Ctrl Pts',(-89.733873976221,-2.31853059017985,-11.6068557395893));
#35442=CARTESIAN_POINT('Ctrl Pts',(-89.6145190716322,3.52938532588192,-11.297744677539));
#35443=CARTESIAN_POINT('Ctrl Pts',(-89.4951641670434,8.51336543905939,-8.22300978186688));
#35444=CARTESIAN_POINT('Ctrl Pts',(-89.3758092624546,11.4133533201776,-3.13539495827318));
#35445=CARTESIAN_POINT('Ctrl Pts',(-89.256454357866,11.5194771350673,2.71974427108801));
#35446=CARTESIAN_POINT('Ctrl Pts',(-89.137099453277,8.80575181376569,7.90911259532042));
#35447=CARTESIAN_POINT('Ctrl Pts',(-89.0177445486884,3.93647217825255,11.1624162917873));
#35448=CARTESIAN_POINT('Ctrl Pts',(-88.8983896440995,-1.89641497438559,
11.6832764729245));
#35449=CARTESIAN_POINT('Ctrl Pts',(-88.7790347395108,-7.26507943176433,
9.34419414546267));
#35450=CARTESIAN_POINT('Ctrl Pts',(-88.659679834922,-10.8553289848437,4.71775104837488));
#35451=CARTESIAN_POINT('Ctrl Pts',(-88.5403249303331,-11.7883081235146,
-1.06354772391229));
#35452=CARTESIAN_POINT('Ctrl Pts',(-88.4209700257445,-9.83563345627059,
-6.58450127641458));
#35453=CARTESIAN_POINT('Ctrl Pts',(-88.3016151211555,-5.47529916018465,
-10.4936381381223));
#35454=CARTESIAN_POINT('Ctrl Pts',(-88.1822602165669,0.225330772320723,
-11.8340427774968));
#35455=CARTESIAN_POINT('Ctrl Pts',(-88.062905311978,5.87080210507991,-10.2775982115417));
#35456=CARTESIAN_POINT('Ctrl Pts',(-87.9435504073893,10.0791628323772,-6.20530571131349));
#35457=CARTESIAN_POINT('Ctrl Pts',(-87.8241955028005,11.8202505156445,-0.61401964082588));
#35458=CARTESIAN_POINT('Ctrl Pts',(-87.7048405982117,10.6678652023627,5.12757197828618));
#35459=CARTESIAN_POINT('Ctrl Pts',(-87.5854856936229,6.90409869651127,9.61398791138743));
#35460=CARTESIAN_POINT('Ctrl Pts',(-87.4661307890342,1.45028144969312,11.7470007272621));
#35461=CARTESIAN_POINT('Ctrl Pts',(-87.3467758844453,-4.35854944134002,
11.0044713247771));
#35462=CARTESIAN_POINT('Ctrl Pts',(-87.2274209798567,-9.10045327408744,
7.56816309128768));
#35463=CARTESIAN_POINT('Ctrl Pts',(-87.1080660752678,-11.6146618674713,
2.2792481379879));
#35464=CARTESIAN_POINT('Ctrl Pts',(-86.988711170679,-11.2857234032786,-3.56760278547595));
#35465=CARTESIAN_POINT('Ctrl Pts',(-86.8693562660902,-8.19415855763303,
-8.54114207249709));
#35466=CARTESIAN_POINT('Ctrl Pts',(-86.7500013615015,-3.0967498864584,-11.423899619261));
#35467=CARTESIAN_POINT('Ctrl Pts',(-86.6306464569127,2.75871058409,-11.5102067002922));
#35468=CARTESIAN_POINT('Ctrl Pts',(-86.5112915523239,7.9388677208545,-8.7789362499679));
#35469=CARTESIAN_POINT('Ctrl Pts',(-86.3919366477351,11.1756735436831,-3.89867454595109));
#35470=CARTESIAN_POINT('Ctrl Pts',(-86.2725817431464,11.6767920331423,1.93594167912407));
#35471=CARTESIAN_POINT('Ctrl Pts',(-86.1532268385575,9.31955465397369,7.29665974414477));
#35472=CARTESIAN_POINT('Ctrl Pts',(-86.0338719339688,4.68098832224899,10.8712322529322));
#35473=CARTESIAN_POINT('Ctrl Pts',(-85.9145170293799,-1.10343471428835,
11.7846414540931));
#35474=CARTESIAN_POINT('Ctrl Pts',(-85.7951621247912,-6.61774853912765,
9.81329438277988));
#35475=CARTESIAN_POINT('Ctrl Pts',(-85.6758072202024,-10.5121071296672,
5.43975606664726));
#35476=CARTESIAN_POINT('Ctrl Pts',(-85.5564523156136,-11.8332124653362,
-0.265377317109467));
#35477=CARTESIAN_POINT('Ctrl Pts',(-85.4370974110249,-10.2576718558679,
-5.90554912498069));
#35478=CARTESIAN_POINT('Ctrl Pts',(-85.3177425064361,-6.17116107030506,
-10.1001046239421));
#35479=CARTESIAN_POINT('Ctrl Pts',(-85.1983876018474,-0.574014965427823,
-11.8222607478303));
#35480=CARTESIAN_POINT('Ctrl Pts',(-85.0790326972585,5.16364396527142,-10.6504517918322));
#35481=CARTESIAN_POINT('Ctrl Pts',(-84.9596777926698,9.63729716650747,-6.87152426282912));
#35482=CARTESIAN_POINT('Ctrl Pts',(-84.8403228880808,11.7518413902604,-1.41051987167687));
#35483=CARTESIAN_POINT('Ctrl Pts',(-84.7209679834923,10.9896584521602,4.39576494765983));
#35484=CARTESIAN_POINT('Ctrl Pts',(-84.6016130789033,7.53732271851852,9.12601274419176));
#35485=CARTESIAN_POINT('Ctrl Pts',(-84.4822581743147,2.23992966389856,11.6223086119325));
#35486=CARTESIAN_POINT('Ctrl Pts',(-84.3629032697258,-3.60577461197105,
11.2735855794793));
#35487=CARTESIAN_POINT('Ctrl Pts',(-84.243548365137,-8.56882318981014,8.16520737717167));
#35488=CARTESIAN_POINT('Ctrl Pts',(-84.1241934605483,-11.4343139809775,
3.05807229378971));
#35489=CARTESIAN_POINT('Ctrl Pts',(-84.0048385559595,-11.5008049803207,
-2.7976467211036));
#35490=CARTESIAN_POINT('Ctrl Pts',(-83.8854836513707,-8.7520198902307,-7.96853124542365));
#35491=CARTESIAN_POINT('Ctrl Pts',(-83.766128746782,-3.86083238868385,-11.1888031369938));
#35492=CARTESIAN_POINT('Ctrl Pts',(-83.6467738421931,1.97544627287577,-11.6701737088792));
#35493=CARTESIAN_POINT('Ctrl Pts',(-83.5274189376044,7.32815646324813,-9.29480850825074));
#35494=CARTESIAN_POINT('Ctrl Pts',(-83.4080640330156,10.8870110362217,-4.64417195135637));
#35495=CARTESIAN_POINT('Ctrl Pts',(-83.2887091284268,11.7808398122987,1.14330905022713));
#35496=CARTESIAN_POINT('Ctrl Pts',(-83.169354223838,9.79084293669987,6.65092002162774));
#35497=CARTESIAN_POINT('Ctrl Pts',(-83.0499993192493,5.40415065493143,10.5304557296806));
#35498=CARTESIAN_POINT('Ctrl Pts',(-82.9306444146604,-0.30542078278036,
11.8322466365892));
#35499=CARTESIAN_POINT('Ctrl Pts',(-82.8112895100717,-5.94022859446243,
10.237628027208));
#35500=CARTESIAN_POINT('Ctrl Pts',(-82.6919346054829,-10.1209305767792,
6.13694575158375));
#35501=CARTESIAN_POINT('Ctrl Pts',(-82.5725797008941,-11.8241359389785,
0.534003724587518));
#35502=CARTESIAN_POINT('Ctrl Pts',(-82.4532247963053,-10.6329156799286,
-5.1996568343135));
#35503=CARTESIAN_POINT('Ctrl Pts',(-82.3338698917166,-6.8388726484708,-9.6604960153945));
#35504=CARTESIAN_POINT('Ctrl Pts',(-82.2145149871277,-1.37073899544396,
-11.7565475443237));
#35505=CARTESIAN_POINT('Ctrl Pts',(-82.095160082539,4.43292358189965,-10.9747195630999));
#35506=CARTESIAN_POINT('Ctrl Pts',(-81.9758051779502,9.15148126279261,-7.50639635738527));
#35507=CARTESIAN_POINT('Ctrl Pts',(-81.8564502733615,11.6297940897892,-2.2005848509751));
#35508=CARTESIAN_POINT('Ctrl Pts',(-81.7370953687727,11.2613771640467,3.64390369531744));
#35509=CARTESIAN_POINT('Ctrl Pts',(-81.6177404641838,8.13604139770176,8.59640893925447));
#35510=CARTESIAN_POINT('Ctrl Pts',(-81.4983855595951,3.01961580316925,11.4445880620795));
#35511=CARTESIAN_POINT('Ctrl Pts',(-81.3790306550063,-2.83705634258411,
11.4912593141579));
#35512=CARTESIAN_POINT('Ctrl Pts',(-81.2994607186138,-6.27653871447523,
9.64670681326287));
#35513=CARTESIAN_POINT('Ctrl Pts',(-81.2596757504175,-7.67112450349791,
8.36830712520962));
#35514=CARTESIAN_POINT('Ctrl Pts',(-90.1653242495824,-5.00646861737615,
10.5068285322322));
#35515=CARTESIAN_POINT('Ctrl Pts',(-90.1255392813862,-6.75744089163788,
9.67249610603002));
#35516=CARTESIAN_POINT('Ctrl Pts',(-90.0459693449937,-9.83227483090726,
7.11203825423161));
#35517=CARTESIAN_POINT('Ctrl Pts',(-89.9266144404048,-12.0382955009232,
1.52736376025392));
#35518=CARTESIAN_POINT('Ctrl Pts',(-89.8072595358161,-11.2970610373474,
-4.43016758299852));
#35519=CARTESIAN_POINT('Ctrl Pts',(-89.6879046312272,-7.79061269803522,
-9.30374792007628));
#35520=CARTESIAN_POINT('Ctrl Pts',(-89.5685497266386,-2.37701312098841,
-11.8996266442545));
#35521=CARTESIAN_POINT('Ctrl Pts',(-89.4491948220497,3.61841041225793,-11.5827185760805));
#35522=CARTESIAN_POINT('Ctrl Pts',(-89.329839917461,8.72810625752566,-8.43042667985563));
#35523=CARTESIAN_POINT('Ctrl Pts',(-89.2104850128721,11.7012433268928,-3.21448204602646));
#35524=CARTESIAN_POINT('Ctrl Pts',(-89.0911301082835,11.8100440050079,2.78834700110977));
#35525=CARTESIAN_POINT('Ctrl Pts',(-88.9717752036945,9.02786777545379,8.10861176215623));
#35526=CARTESIAN_POINT('Ctrl Pts',(-88.8524202991058,4.03576560850392,11.4439766720762));
#35527=CARTESIAN_POINT('Ctrl Pts',(-88.7330653945171,-1.94425007633985,
11.9779750113724));
#35528=CARTESIAN_POINT('Ctrl Pts',(-88.6137104899282,-7.44833352963752,
9.57989175683245));
#35529=CARTESIAN_POINT('Ctrl Pts',(-88.4943555853395,-11.1291434061337,
4.83675142827165));
#35530=CARTESIAN_POINT('Ctrl Pts',(-88.3750006807507,-12.0856559764755,
-1.09037461280197));
#35531=CARTESIAN_POINT('Ctrl Pts',(-88.2556457761619,-10.0837271148422,
-6.75058849578874));
#35532=CARTESIAN_POINT('Ctrl Pts',(-88.1362908715731,-5.61340790594708,
-10.7583292827231));
#35533=CARTESIAN_POINT('Ctrl Pts',(-88.0169359669844,0.231014507480469,
-12.1325442396971));
#35534=CARTESIAN_POINT('Ctrl Pts',(-87.8975810623955,6.01888700265922,-10.5368399729359));
#35535=CARTESIAN_POINT('Ctrl Pts',(-87.7782261578068,10.3333992670249,-6.36182811562228));
#35536=CARTESIAN_POINT('Ctrl Pts',(-87.658871253218,12.1184040823362,-0.629507649788865));
#35537=CARTESIAN_POINT('Ctrl Pts',(-87.5395163486293,10.9369510440597,5.25690966633021));
#35538=CARTESIAN_POINT('Ctrl Pts',(-87.4201614440405,7.07824742952097,9.85649079084144));
#35539=CARTESIAN_POINT('Ctrl Pts',(-87.3008065394516,1.48686329593746,12.0433066439708));
#35540=CARTESIAN_POINT('Ctrl Pts',(-87.181451634863,-4.46848933303842,11.2820477069948));
#35541=CARTESIAN_POINT('Ctrl Pts',(-87.0620967302741,-9.33000277463225,
7.75906216030367));
#35542=CARTESIAN_POINT('Ctrl Pts',(-86.9427418256853,-11.9076296736208,
2.33673980965908));
#35543=CARTESIAN_POINT('Ctrl Pts',(-86.8233869210965,-11.5703940776379,
-3.65759186765497));
#35544=CARTESIAN_POINT('Ctrl Pts',(-86.7040320165078,-8.4008477133969,-8.75658352774929));
#35545=CARTESIAN_POINT('Ctrl Pts',(-86.584677111919,-3.17486219233364,-11.7120556454386));
#35546=CARTESIAN_POINT('Ctrl Pts',(-86.4653222073302,2.82829619896576,-11.8005397331251));
#35547=CARTESIAN_POINT('Ctrl Pts',(-86.3459673027414,8.1391174298885,-9.00037581685552));
#35548=CARTESIAN_POINT('Ctrl Pts',(-86.2266123981526,11.4575683244089,-3.9970145701077));
#35549=CARTESIAN_POINT('Ctrl Pts',(-86.1072574935638,11.9713270083183,1.984773801233));
#35550=CARTESIAN_POINT('Ctrl Pts',(-85.9879025889751,9.55463075971132,7.48071042266241));
#35551=CARTESIAN_POINT('Ctrl Pts',(-85.8685476843863,4.79906140048653,11.1454478176748));
#35552=CARTESIAN_POINT('Ctrl Pts',(-85.7491927797975,-1.13126771116443,
12.0818968191186));
#35553=CARTESIAN_POINT('Ctrl Pts',(-85.6298378752088,-6.78467438624051,
10.0608245613788));
#35554=CARTESIAN_POINT('Ctrl Pts',(-85.5104829706199,-10.7772641354352,
5.57696827471827));
#35555=CARTESIAN_POINT('Ctrl Pts',(-85.3911280660311,-12.1316929837729,
-0.272071184850303));
#35556=CARTESIAN_POINT('Ctrl Pts',(-85.2717731614424,-10.5164109955954,
-6.05451048011913));
#35557=CARTESIAN_POINT('Ctrl Pts',(-85.1524182568537,-6.32682221143786,
-10.3548692935743));
#35558=CARTESIAN_POINT('Ctrl Pts',(-85.0330633522648,-0.588493897921702,
-12.1204650205452));
#35559=CARTESIAN_POINT('Ctrl Pts',(-84.913708447676,5.29389153179587,-10.9190983982988));
#35560=CARTESIAN_POINT('Ctrl Pts',(-84.7943535430873,9.88038799776011,-7.044851339515));
#35561=CARTESIAN_POINT('Ctrl Pts',(-84.6749986384985,12.0482694076755,-1.44609877333157));
#35562=CARTESIAN_POINT('Ctrl Pts',(-84.5556437339097,11.2668611950207,4.50664356192851));
#35563=CARTESIAN_POINT('Ctrl Pts',(-84.4362888293209,7.72744387109975,9.35620695587567));
#35564=CARTESIAN_POINT('Ctrl Pts',(-84.3169339247322,2.29642956781735,11.9154692992846));
#35565=CARTESIAN_POINT('Ctrl Pts',(-84.1975790201435,-3.69672653890549,
11.557950089815));
#35566=CARTESIAN_POINT('Ctrl Pts',(-84.0782241155545,-8.78496287255304,
8.37116626941845));
#35567=CARTESIAN_POINT('Ctrl Pts',(-83.9588692109658,-11.7227326986341,
3.13520899748206));
#35568=CARTESIAN_POINT('Ctrl Pts',(-83.839514306377,-11.7909008645129,-2.86821445967534));
#35569=CARTESIAN_POINT('Ctrl Pts',(-83.7201594017883,-8.97278051984475,
-8.16952918611646));
#35570=CARTESIAN_POINT('Ctrl Pts',(-83.6008044971995,-3.9582178836496,-11.4710290981011));
#35571=CARTESIAN_POINT('Ctrl Pts',(-83.4814495926107,2.02527485741264,-11.964541743686));
#35572=CARTESIAN_POINT('Ctrl Pts',(-83.3620946880219,7.51300161385648,-9.52926041811373));
#35573=CARTESIAN_POINT('Ctrl Pts',(-83.2427397834331,11.1616246044169,-4.76131637480104));
#35574=CARTESIAN_POINT('Ctrl Pts',(-83.1233848788443,12.0779992848507,1.17214783589458));
#35575=CARTESIAN_POINT('Ctrl Pts',(-83.0040299742556,10.0378068008441,6.81868258500195));
#35576=CARTESIAN_POINT('Ctrl Pts',(-82.8846750696668,5.54046475339955,10.7960755598643));
#35577=CARTESIAN_POINT('Ctrl Pts',(-82.7653201650779,-0.313124705434724,
12.1307027929969));
#35578=CARTESIAN_POINT('Ctrl Pts',(-82.6459652604893,-6.09006470327072,
10.4958615821344));
#35579=CARTESIAN_POINT('Ctrl Pts',(-82.5266103559004,-10.3762205594841,
6.2917438467685));
#35580=CARTESIAN_POINT('Ctrl Pts',(-82.4072554513117,-12.1223875114463,
0.547473415005821));
#35581=CARTESIAN_POINT('Ctrl Pts',(-82.2879005467229,-10.9011199561499,
-5.33081278812953));
#35582=CARTESIAN_POINT('Ctrl Pts',(-82.1685456421341,-7.01137612203031,
-9.90417201356299));
#35583=CARTESIAN_POINT('Ctrl Pts',(-82.0491907375453,-1.40531446573152,
-12.0530942695968));
#35584=CARTESIAN_POINT('Ctrl Pts',(-81.9298358329565,4.54473948419936,-11.2515454879692));
#35585=CARTESIAN_POINT('Ctrl Pts',(-81.8104809283678,9.38231789145822,-7.69573742456438));
#35586=CARTESIAN_POINT('Ctrl Pts',(-81.6911260237789,11.9231435905609,-2.25609232277172));
#35587=CARTESIAN_POINT('Ctrl Pts',(-81.5717711191902,11.5454337297581,3.73581738885568));
#35588=CARTESIAN_POINT('Ctrl Pts',(-81.4524162146014,8.34126460834911,8.81324444393242));
#35589=CARTESIAN_POINT('Ctrl Pts',(-81.3330613100126,3.0957824817487,11.733265932782));
#35590=CARTESIAN_POINT('Ctrl Pts',(-81.2137064054238,-2.9086181480067,11.7811144188159));
#35591=CARTESIAN_POINT('Ctrl Pts',(-81.1341364690313,-6.43485789745049,
9.89003499310112));
#35592=CARTESIAN_POINT('Ctrl Pts',(-81.0943515008351,-7.86462066740977,
8.57938899807272));
#35593=CARTESIAN_POINT('Ctrl Pts',(-90.,-5.12964461189318,10.765331911078));
#35594=CARTESIAN_POINT('Ctrl Pts',(-89.9602150318037,-6.92369670303529,
9.91047209636926));
#35595=CARTESIAN_POINT('Ctrl Pts',(-89.8806450954113,-10.0741819161646,
7.2870183553687));
#35596=CARTESIAN_POINT('Ctrl Pts',(-89.7612901908224,-12.3344781266306,
1.56494205436438));
#35597=CARTESIAN_POINT('Ctrl Pts',(-89.6419352862337,-11.5750067980709,
-4.53916463054197));
#35598=CARTESIAN_POINT('Ctrl Pts',(-89.5225803816448,-7.98228801657151,
-9.5326514627478));
#35599=CARTESIAN_POINT('Ctrl Pts',(-89.4032254770562,-2.43549565179697,
-12.1923975489198));
#35600=CARTESIAN_POINT('Ctrl Pts',(-89.2838705724673,3.70743549863393,-11.8676924746221));
#35601=CARTESIAN_POINT('Ctrl Pts',(-89.1645156678785,8.94284707599193,-8.63784357784438));
#35602=CARTESIAN_POINT('Ctrl Pts',(-89.0451607632897,11.989133333608,-3.29356913377973));
#35603=CARTESIAN_POINT('Ctrl Pts',(-88.925805858701,12.1006108749485,2.85694973113152));
#35604=CARTESIAN_POINT('Ctrl Pts',(-88.8064509541121,9.24998373714189,8.30811092899203));
#35605=CARTESIAN_POINT('Ctrl Pts',(-88.6870960495233,4.13505903875529,11.7255370523651));
#35606=CARTESIAN_POINT('Ctrl Pts',(-88.5677411449347,-1.9920851782941,12.2726735498203));
#35607=CARTESIAN_POINT('Ctrl Pts',(-88.4483862403458,-7.63158762751069,
9.81558936820223));
#35608=CARTESIAN_POINT('Ctrl Pts',(-88.3290313357571,-11.4029578274237,
4.95575180816843));
#35609=CARTESIAN_POINT('Ctrl Pts',(-88.2096764311682,-12.3830038294364,
-1.11720150169165));
#35610=CARTESIAN_POINT('Ctrl Pts',(-88.0903215265795,-10.3318207734139,
-6.9166757151629));
#35611=CARTESIAN_POINT('Ctrl Pts',(-87.9709666219907,-5.75151665170952,
-11.0230204273238));
#35612=CARTESIAN_POINT('Ctrl Pts',(-87.8516117174019,0.236698242640219,
-12.4310457018974));
#35613=CARTESIAN_POINT('Ctrl Pts',(-87.7322568128131,6.16697190023853,-10.79608173433));
#35614=CARTESIAN_POINT('Ctrl Pts',(-87.6129019082243,10.5876357016726,-6.51835051993107));
#35615=CARTESIAN_POINT('Ctrl Pts',(-87.4935470036357,12.416557649028,-0.644995658751849));
#35616=CARTESIAN_POINT('Ctrl Pts',(-87.3741920990467,11.2060368857567,5.38624735437424));
#35617=CARTESIAN_POINT('Ctrl Pts',(-87.2548371944581,7.25239616253066,10.0989936702955));
#35618=CARTESIAN_POINT('Ctrl Pts',(-87.1354822898692,1.52344514218181,12.3396125606794));
#35619=CARTESIAN_POINT('Ctrl Pts',(-87.0161273852805,-4.57842922473682,
11.5596240892125));
#35620=CARTESIAN_POINT('Ctrl Pts',(-86.8967724806917,-9.55955227517707,
7.94996122931966));
#35621=CARTESIAN_POINT('Ctrl Pts',(-86.7774175761029,-12.2005974797702,
2.39423148133028));
#35622=CARTESIAN_POINT('Ctrl Pts',(-86.6580626715141,-11.8550647519971,
-3.74758094983401));
#35623=CARTESIAN_POINT('Ctrl Pts',(-86.5387077669254,-8.60753686916077,
-8.97202498300148));
#35624=CARTESIAN_POINT('Ctrl Pts',(-86.4193528623365,-3.25297449820887,
-12.0002116716161));
#35625=CARTESIAN_POINT('Ctrl Pts',(-86.2999979577478,2.89788181384153,-12.090872765958));
#35626=CARTESIAN_POINT('Ctrl Pts',(-86.1806430531589,8.3393671389225,-9.22181538374314));
#35627=CARTESIAN_POINT('Ctrl Pts',(-86.0612881485703,11.7394631051347,-4.09535459426431));
#35628=CARTESIAN_POINT('Ctrl Pts',(-85.9419332439813,12.2658619834943,2.03360592334192));
#35629=CARTESIAN_POINT('Ctrl Pts',(-85.8225783393927,9.78970686544896,7.66476110118005));
#35630=CARTESIAN_POINT('Ctrl Pts',(-85.7032234348038,4.91713447872407,11.4196633824174));
#35631=CARTESIAN_POINT('Ctrl Pts',(-85.5838685302151,-1.15910070804053,
12.3791521841442));
#35632=CARTESIAN_POINT('Ctrl Pts',(-85.4645136256264,-6.95160023335335,
10.3083547399778));
#35633=CARTESIAN_POINT('Ctrl Pts',(-85.3451587210375,-11.0424211412032,
5.71418048278927));
#35634=CARTESIAN_POINT('Ctrl Pts',(-85.2258038164488,-12.4301735022096,
-0.278765052591136));
#35635=CARTESIAN_POINT('Ctrl Pts',(-85.1064489118599,-10.7751501353228,
-6.20347183525758));
#35636=CARTESIAN_POINT('Ctrl Pts',(-84.9870940072712,-6.48248335257065,
-10.6096339632065));
#35637=CARTESIAN_POINT('Ctrl Pts',(-84.8677391026824,-0.602972830415581,
-12.4186692932601));
#35638=CARTESIAN_POINT('Ctrl Pts',(-84.7483841980936,5.42413909832031,-11.1877450047655));
#35639=CARTESIAN_POINT('Ctrl Pts',(-84.6290292935049,10.1234788290128,-7.21817841620088));
#35640=CARTESIAN_POINT('Ctrl Pts',(-84.509674388916,12.3446974250905,-1.48167767498628));
#35641=CARTESIAN_POINT('Ctrl Pts',(-84.3903194843273,11.5440639378813,4.6175221761972));
#35642=CARTESIAN_POINT('Ctrl Pts',(-84.2709645797385,7.91756502368096,9.58640116755958));
#35643=CARTESIAN_POINT('Ctrl Pts',(-84.1516096751497,2.35292947173615,12.2086299866367));
#35644=CARTESIAN_POINT('Ctrl Pts',(-84.032254770561,-3.78767846583993,11.8423146001506));
#35645=CARTESIAN_POINT('Ctrl Pts',(-83.9128998659722,-9.00110255529593,
8.57712516166523));
#35646=CARTESIAN_POINT('Ctrl Pts',(-83.7935449613833,-12.0111514162906,
3.21234570117441));
#35647=CARTESIAN_POINT('Ctrl Pts',(-83.6741900567945,-12.0809967487051,
-2.93878219824708));
#35648=CARTESIAN_POINT('Ctrl Pts',(-83.5548351522058,-9.1935411494588,-8.37052712680928));
#35649=CARTESIAN_POINT('Ctrl Pts',(-83.435480247617,-4.05560337861534,-11.7532550592084));
#35650=CARTESIAN_POINT('Ctrl Pts',(-83.3161253430283,2.07510344194952,-12.2589097784928));
#35651=CARTESIAN_POINT('Ctrl Pts',(-83.1967704384394,7.69784676446482,-9.7637123279767));
#35652=CARTESIAN_POINT('Ctrl Pts',(-83.0774155338507,11.4362381726121,-4.87846079824571));
#35653=CARTESIAN_POINT('Ctrl Pts',(-82.9580606292618,12.3751587574026,1.20098662156203));
#35654=CARTESIAN_POINT('Ctrl Pts',(-82.8387057246731,10.2847706649882,6.98644514837616));
#35655=CARTESIAN_POINT('Ctrl Pts',(-82.7193508200843,5.67677885186767,11.0616953900479));
#35656=CARTESIAN_POINT('Ctrl Pts',(-82.5999959154955,-0.320828628089087,
12.4291589494046));
#35657=CARTESIAN_POINT('Ctrl Pts',(-82.4806410109069,-6.23990081207901,
10.7540951370608));
#35658=CARTESIAN_POINT('Ctrl Pts',(-82.361286106318,-10.631510542189,6.44654194195327));
#35659=CARTESIAN_POINT('Ctrl Pts',(-82.2419312017292,-12.4206390839141,
0.560943105424116));
#35660=CARTESIAN_POINT('Ctrl Pts',(-82.1225762971405,-11.1693242323713,
-5.46196874194555));
#35661=CARTESIAN_POINT('Ctrl Pts',(-82.0032213925516,-7.18387959558981,
-10.1478480117315));
#35662=CARTESIAN_POINT('Ctrl Pts',(-81.8838664879629,-1.43988993601907,
-12.3496409948698));
#35663=CARTESIAN_POINT('Ctrl Pts',(-81.764511583374,4.65655538649907,-11.5283714128385));
#35664=CARTESIAN_POINT('Ctrl Pts',(-81.6451566787854,9.61315452012383,-7.88507849174348));
#35665=CARTESIAN_POINT('Ctrl Pts',(-81.5258017741965,12.2164930913327,-2.31159979456833));
#35666=CARTESIAN_POINT('Ctrl Pts',(-81.4064468696078,11.8294902954694,3.82773108239391));
#35667=CARTESIAN_POINT('Ctrl Pts',(-81.287091965019,8.54648781899647,9.03007994861038));
#35668=CARTESIAN_POINT('Ctrl Pts',(-81.1677370604302,3.17194916032815,12.0219438034846));
#35669=CARTESIAN_POINT('Ctrl Pts',(-81.0483821558414,-2.9801799534293,12.0709695234739));
#35670=CARTESIAN_POINT('Ctrl Pts',(-80.9688122194489,-6.59317708042574,
10.1333631729394));
#35671=CARTESIAN_POINT('Ctrl Pts',(-80.9290272512526,-8.05811683132163,
8.79047087093582));
#35672=CARTESIAN_POINT('Ctrl Pts',(-82.2311568471519,-11.9258224962353,
0.000178908662697473));
#35673=CARTESIAN_POINT('Ctrl Pts',(-82.1949633304814,-11.92451531224,-1.80734341106785));
#35674=CARTESIAN_POINT('Ctrl Pts',(-82.1587698138109,-11.5076407664426,
-3.6154480232762));
#35675=CARTESIAN_POINT('Ctrl Pts',(-82.1225762971404,-10.7136359348315,
-5.23912997901492));
#35676=CARTESIAN_POINT('Ctrl Pts',(-82.0827913289442,-9.84084268677745,
-7.02392849854086));
#35677=CARTESIAN_POINT('Ctrl Pts',(-82.0430063607478,-8.51236114118363,
-8.58588825513617));
#35678=CARTESIAN_POINT('Ctrl Pts',(-82.0032213925516,-6.89078875845827,
-9.73383363062355));
#35679=CARTESIAN_POINT('Ctrl Pts',(-81.9634364243553,-5.2692163757329,-10.8817790061109));
#35680=CARTESIAN_POINT('Ctrl Pts',(-81.9236514561591,-3.35455315587599,
-11.6157100004904));
#35681=CARTESIAN_POINT('Ctrl Pts',(-81.8838664879629,-1.38114732552784,
-11.8457972340082));
#35682=CARTESIAN_POINT('Ctrl Pts',(-81.8440815197666,0.592258504820307,
-12.075884467526));
#35683=CARTESIAN_POINT('Ctrl Pts',(-81.8042965515703,2.62440694565969,-11.8021279401822));
#35684=CARTESIAN_POINT('Ctrl Pts',(-81.7645115833741,4.46658102168351,-11.0580341896612));
#35685=CARTESIAN_POINT('Ctrl Pts',(-81.7247266151778,6.30875509770729,-10.3139404391402));
#35686=CARTESIAN_POINT('Ctrl Pts',(-81.6849416469816,7.96095480891553,-9.09950946544184));
#35687=CARTESIAN_POINT('Ctrl Pts',(-81.6451566787853,9.22094442638779,-7.56338086239685));
#35688=CARTESIAN_POINT('Ctrl Pts',(-81.6053717105891,10.4809340438601,-6.02725225935181));
#35689=CARTESIAN_POINT('Ctrl Pts',(-81.5655867423928,11.3487135675964,-4.16942602696006));
#35690=CARTESIAN_POINT('Ctrl Pts',(-81.5258017741965,11.7181028634873,-2.21729109793712));
#35691=CARTESIAN_POINT('Ctrl Pts',(-81.4922011827977,12.0300724178455,-0.568605901509375));
#35692=CARTESIAN_POINT('Ctrl Pts',(-81.4586005913988,11.9865536565682,1.14734714617648));
#35693=CARTESIAN_POINT('Ctrl Pts',(-81.425,11.5970184578307,2.77968392481168));
#35694=CARTESIAN_POINT('Ctrl Pts',(-90.,-6.42475130859185,-9.01043996637154));
#35695=CARTESIAN_POINT('Ctrl Pts',(-89.9663994086011,-5.15589024403101,
-9.91327621792232));
#35696=CARTESIAN_POINT('Ctrl Pts',(-89.8930138490061,-1.9646812879697,-11.2984722410166));
#35697=CARTESIAN_POINT('Ctrl Pts',(-89.7798433212146,3.44036023950592,-11.0127707789974));
#35698=CARTESIAN_POINT('Ctrl Pts',(-89.6604884166259,8.29862462059312,-8.01559288387814));
#35699=CARTESIAN_POINT('Ctrl Pts',(-89.5411335120371,11.1254633134624,-3.0563078705199));
#35700=CARTESIAN_POINT('Ctrl Pts',(-89.4217786074483,11.2289102651267,2.65114154106624));
#35701=CARTESIAN_POINT('Ctrl Pts',(-89.3024237028595,8.5836358520776,7.70961342848463));
#35702=CARTESIAN_POINT('Ctrl Pts',(-89.1830687982707,3.83717874800117,10.8808559114985));
#35703=CARTESIAN_POINT('Ctrl Pts',(-89.063713893682,-1.84857987243133,11.3885779344766));
#35704=CARTESIAN_POINT('Ctrl Pts',(-88.9443589890932,-7.08182533389115,
9.10849653409288));
#35705=CARTESIAN_POINT('Ctrl Pts',(-88.8321642231656,-10.3715670943498,
4.8692917563021));
#35706=CARTESIAN_POINT('Ctrl Pts',(-88.7597544254343,-11.0647130263883,
1.51184016271179));
#35707=CARTESIAN_POINT('Ctrl Pts',(-88.7271295958992,-11.0662550916496,
-0.000269981886922149));
#35708=CARTESIAN_POINT('Origin',(-92.7728704041008,0.,0.));
#35709=CARTESIAN_POINT('Ctrl Pts',(-90.,6.42428395783973,-9.01020671414053));
#35710=CARTESIAN_POINT('Ctrl Pts',(-89.9602150318037,7.92584288148909,-7.93959410657265));
#35711=CARTESIAN_POINT('Ctrl Pts',(-89.8806450954112,10.3816473609839,-5.03396371914769));
#35712=CARTESIAN_POINT('Ctrl Pts',(-89.7612901908224,11.5241044785577,0.559683279179561));
#35713=CARTESIAN_POINT('Ctrl Pts',(-89.6419352862336,9.84536941628095,6.01529970711026));
#35714=CARTESIAN_POINT('Ctrl Pts',(-89.5225803816449,5.75668384652155,9.99893950199032));
#35715=CARTESIAN_POINT('Ctrl Pts',(-89.4032254770561,0.258777053280351,
11.5347028377517));
#35716=CARTESIAN_POINT('Ctrl Pts',(-89.2838705724674,-5.30245378001128,
10.2470084955505));
#35717=CARTESIAN_POINT('Ctrl Pts',(-89.1645156678784,-9.56571023252816,
6.45089830374292));
#35718=CARTESIAN_POINT('Ctrl Pts',(-89.0775156117564,-10.9664491639747,
2.53281638713329));
#35719=CARTESIAN_POINT('Ctrl Pts',(-89.0303005238305,-11.0665694714916,
0.344653378612825));
#35720=CARTESIAN_POINT('Ctrl Pts',(-89.0228704041008,-11.0662155972561,
0.000275354078309552));
#35721=CARTESIAN_POINT('Ctrl Pts',(-90.4959727487473,6.9230012965212,-9.70966930684902));
#35722=CARTESIAN_POINT('Ctrl Pts',(-90.4561877805511,8.54112628032454,-8.55594501338601));
#35723=CARTESIAN_POINT('Ctrl Pts',(-90.3766178441585,11.1875749284727,-5.4247504598192));
#35724=CARTESIAN_POINT('Ctrl Pts',(-90.2572629395698,12.4187210232109,0.603131507391253));
#35725=CARTESIAN_POINT('Ctrl Pts',(-90.137908034981,10.6096657123112,6.48226758726452));
#35726=CARTESIAN_POINT('Ctrl Pts',(-90.0185531303922,6.20357537037213,10.7751574479583));
#35727=CARTESIAN_POINT('Ctrl Pts',(-89.8991982258034,0.278865922977081,
12.4301421333179));
#35728=CARTESIAN_POINT('Ctrl Pts',(-89.7798433212147,-5.71408341142283,
11.0424840442474));
#35729=CARTESIAN_POINT('Ctrl Pts',(-89.6604884166258,-10.3082965785042,
6.95168171482198));
#35730=CARTESIAN_POINT('Ctrl Pts',(-89.5411335120371,-12.3791417069743,
1.15920985029086));
#35731=CARTESIAN_POINT('Ctrl Pts',(-89.4217786074483,-11.4197057842347,
-4.9170383670988));
#35732=CARTESIAN_POINT('Ctrl Pts',(-89.3024237028595,-7.66484473635443,
-9.78964058399421));
#35733=CARTESIAN_POINT('Ctrl Pts',(-89.1830687982707,-2.0337109283889,-12.2658449959716));
#35734=CARTESIAN_POINT('Ctrl Pts',(-89.0637138936819,4.09525421691159,-11.7394980107209));
#35735=CARTESIAN_POINT('Ctrl Pts',(-88.9443589890932,9.22174406413998,-8.33944614371624));
#35736=CARTESIAN_POINT('Ctrl Pts',(-88.8250040845043,12.0908480304004,-2.89798521694021));
#35737=CARTESIAN_POINT('Ctrl Pts',(-88.7056491799157,12.0002395423682,3.25287183483145));
#35738=CARTESIAN_POINT('Ctrl Pts',(-88.5862942753267,8.97209865335899,8.60746016016937));
#35739=CARTESIAN_POINT('Ctrl Pts',(-88.4669393707381,3.74768237847767,11.8550327346267));
#35740=CARTESIAN_POINT('Ctrl Pts',(-88.3475844661492,-2.39412711940671,
12.2006180109483));
#35741=CARTESIAN_POINT('Ctrl Pts',(-88.2282295615605,-7.94987948258836,
9.55962031973835));
#35742=CARTESIAN_POINT('Ctrl Pts',(-88.1088746569717,-11.559584967541,4.57852813059656));
#35743=CARTESIAN_POINT('Ctrl Pts',(-87.9895197523829,-12.3396256411026,
-1.52333958832352));
#35744=CARTESIAN_POINT('Ctrl Pts',(-87.8701648477942,-10.0990557505557,
-7.25230979806363));
#35745=CARTESIAN_POINT('Ctrl Pts',(-87.7508099432053,-5.38634323820261,
-11.2059908523829));
#35746=CARTESIAN_POINT('Ctrl Pts',(-87.6314550386166,0.644889443233899,
-12.4165632148108));
#35747=CARTESIAN_POINT('Ctrl Pts',(-87.5121001340277,6.51825997214534,-10.5876915046587));
#35748=CARTESIAN_POINT('Ctrl Pts',(-87.3927452294391,10.796029021505,-6.16706427960833));
#35749=CARTESIAN_POINT('Ctrl Pts',(-87.2733903248502,12.4310437232692,-0.236804586541372));
#35750=CARTESIAN_POINT('Ctrl Pts',(-87.1540354202615,11.0230696761805,5.75142237852022));
#35751=CARTESIAN_POINT('Ctrl Pts',(-87.0346805156726,6.91676411733848,10.3317616410336));
#35752=CARTESIAN_POINT('Ctrl Pts',(-86.9153256110839,1.11730745581452,12.3829943273524));
#35753=CARTESIAN_POINT('Ctrl Pts',(-86.7959707064951,-4.95565431861441,
11.4030002515323));
#35754=CARTESIAN_POINT('Ctrl Pts',(-86.6766158019064,-9.81552404136514,
7.63167165537372));
#35755=CARTESIAN_POINT('Ctrl Pts',(-86.5572608973175,-12.2726567223273,
1.99219011089958));
#35756=CARTESIAN_POINT('Ctrl Pts',(-86.4379059927288,-11.7255721262879,
-4.13495861808445));
#35757=CARTESIAN_POINT('Ctrl Pts',(-86.31855108814,-8.30819080790685,-9.24991297048049));
#35758=CARTESIAN_POINT('Ctrl Pts',(-86.1991961835512,-2.85705176856468,
-12.100585921921));
#35759=CARTESIAN_POINT('Ctrl Pts',(-86.0798412789625,3.29346349212934,-11.9891627183912));
#35760=CARTESIAN_POINT('Ctrl Pts',(-85.9604863743736,8.63777353189284,-8.94291858812224));
#35761=CARTESIAN_POINT('Ctrl Pts',(-85.8411314697849,11.867647466544,-3.70754205261153));
#35762=CARTESIAN_POINT('Ctrl Pts',(-85.7217765651961,12.192446129963,2.43540177999482));
#35763=CARTESIAN_POINT('Ctrl Pts',(-85.6024216606073,9.53266222570474,7.98218487337101));
#35764=CARTESIAN_POINT('Ctrl Pts',(-85.4830667560185,4.53938287687979,11.575013069502));
#35765=CARTESIAN_POINT('Ctrl Pts',(-85.3637118514297,-1.56508965319305,
12.3343998167531));
#35766=CARTESIAN_POINT('Ctrl Pts',(-85.244356946841,-7.28644469839213,10.0744552269254));
#35767=CARTESIAN_POINT('Ctrl Pts',(-85.1250020422522,-11.224154723112,5.34838996462391));
#35768=CARTESIAN_POINT('Ctrl Pts',(-85.0056471376634,-12.4143097316831,
-0.686904904551077));
#35769=CARTESIAN_POINT('Ctrl Pts',(-84.8862922330746,-10.5655722965231,
-6.55405267822735));
#35770=CARTESIAN_POINT('Ctrl Pts',(-84.7669373284858,-6.13049389601684,
-10.8168372943746));
#35771=CARTESIAN_POINT('Ctrl Pts',(-84.6475824238971,-0.194735072702333,
-12.4317739166017));
#35772=CARTESIAN_POINT('Ctrl Pts',(-84.5282275193082,5.78869284809667,-11.003543046328));
#35773=CARTESIAN_POINT('Ctrl Pts',(-84.4088726147195,10.3551096474539,-6.88176057789721));
#35774=CARTESIAN_POINT('Ctrl Pts',(-84.2895177101307,12.3867045241691,-1.07539550506673));
#35775=CARTESIAN_POINT('Ctrl Pts',(-84.1701628055419,11.3861644217084,4.99421507598957));
#35776=CARTESIAN_POINT('Ctrl Pts',(-84.0508079009532,7.59841103272048,9.84129433752252));
#35777=CARTESIAN_POINT('Ctrl Pts',(-83.9314529963644,1.95064654649944,12.2793282599065));
#35778=CARTESIAN_POINT('Ctrl Pts',(-83.8120980917756,-4.17461569768676,
11.7115117829036));
#35779=CARTESIAN_POINT('Ctrl Pts',(-83.6927431871868,-9.27797592714853,
8.27684040805947));
#35780=CARTESIAN_POINT('Ctrl Pts',(-83.573388282598,-12.1101852435648,2.81608555969103));
#35781=CARTESIAN_POINT('Ctrl Pts',(-83.4540333780092,-11.9779485826422,
-3.33401741156248));
#35782=CARTESIAN_POINT('Ctrl Pts',(-83.3346784734205,-8.91363611698198,
-8.66798799194735));
#35783=CARTESIAN_POINT('Ctrl Pts',(-83.2153235688317,-3.66735924645335,
-11.8801262790221));
#35784=CARTESIAN_POINT('Ctrl Pts',(-83.0959686642429,2.47664850863613,-12.1841346256725));
#35785=CARTESIAN_POINT('Ctrl Pts',(-82.9766137596541,8.01439893416919,-9.50559494678961));
#35786=CARTESIAN_POINT('Ctrl Pts',(-82.8572588550654,11.5903084357114,-4.50018566393989));
#35787=CARTESIAN_POINT('Ctrl Pts',(-82.7379039504766,12.3290330986776,1.60682184985248));
#35788=CARTESIAN_POINT('Ctrl Pts',(-82.6185490458878,10.0497385722665,7.32049603683421));
#35789=CARTESIAN_POINT('Ctrl Pts',(-82.499194141299,5.31037700842289,11.2421902906159));
#35790=CARTESIAN_POINT('Ctrl Pts',(-82.3798392367102,-0.728915757906636,
12.4119135791479));
#35791=CARTESIAN_POINT('Ctrl Pts',(-82.2604843321214,-6.58976355633953,
10.5433331203244));
#35792=CARTESIAN_POINT('Ctrl Pts',(-82.1411294275327,-10.8375357501615,
6.09385116031955));
#35793=CARTESIAN_POINT('Ctrl Pts',(-82.0217745229439,-12.4323325327718,
0.152667783329525));
#35794=CARTESIAN_POINT('Ctrl Pts',(-81.9024196183551,-10.9839510962759,
-5.82590625729596));
#35795=CARTESIAN_POINT('Ctrl Pts',(-81.7830647137663,-6.84655244795005,
-10.3783196702241));
#35796=CARTESIAN_POINT('Ctrl Pts',(-81.6637098091776,-1.03373760445683,
-12.390310166928));
#35797=CARTESIAN_POINT('Ctrl Pts',(-81.5443549045887,5.03323825502514,-11.3690924439751));
#35798=CARTESIAN_POINT('Ctrl Pts',(-81.4647849681962,8.25438701496757,-8.83290032863896));
#35799=CARTESIAN_POINT('Ctrl Pts',(-81.425,9.46357049537284,-7.25578792958482));
#35800=CARTESIAN_POINT('Ctrl Pts',(-90.3306484991649,6.75676218362737,-9.47651510927952));
#35801=CARTESIAN_POINT('Ctrl Pts',(-90.2908635309686,8.33603181404606,-8.35049471111489));
#35802=CARTESIAN_POINT('Ctrl Pts',(-90.2112935945761,10.9189324059764,-5.2944882129287));
#35803=CARTESIAN_POINT('Ctrl Pts',(-90.0919386899874,12.1205155083265,0.588648764654024));
#35804=CARTESIAN_POINT('Ctrl Pts',(-89.9725837853985,10.3549002803011,6.3266116272131));
#35805=CARTESIAN_POINT('Ctrl Pts',(-89.8532288808098,6.0546115290886,10.5164181326357));
#35806=CARTESIAN_POINT('Ctrl Pts',(-89.733873976221,0.272169633078173,12.1316623681291));
#35807=CARTESIAN_POINT('Ctrl Pts',(-89.6145190716323,-5.57687353428564,
10.7773255280151));
#35808=CARTESIAN_POINT('Ctrl Pts',(-89.4951641670433,-10.0607677965122,
6.78475391112896));
#35809=CARTESIAN_POINT('Ctrl Pts',(-89.3758092624547,-12.0818865935326,
1.1313742326279));
#35810=CARTESIAN_POINT('Ctrl Pts',(-89.2564543578658,-11.1454892013152,
-4.79896759674922));
#35811=CARTESIAN_POINT('Ctrl Pts',(-89.1370994532771,-7.48079204954058,
-9.55456606984521));
#35812=CARTESIAN_POINT('Ctrl Pts',(-89.0177445486883,-1.98487628483803,
-11.9713104287099));
#35813=CARTESIAN_POINT('Ctrl Pts',(-88.8983896440995,3.99691660307405,-11.457602391822));
#35814=CARTESIAN_POINT('Ctrl Pts',(-88.7790347395108,9.00030620981994,-8.13919453757342));
#35815=CARTESIAN_POINT('Ctrl Pts',(-88.6596798349219,11.8005155915321,-2.8283971190894));
#35816=CARTESIAN_POINT('Ctrl Pts',(-88.5403249303332,11.712082846942,3.17476199416864));
#35817=CARTESIAN_POINT('Ctrl Pts',(-88.4209700257444,8.75665542909154,8.40077284638618));
#35818=CARTESIAN_POINT('Ctrl Pts',(-88.3016151211556,3.65769086073536,11.570362829087));
#35819=CARTESIAN_POINT('Ctrl Pts',(-88.1822602165668,-2.33663795373441,
11.9076497117923));
#35820=CARTESIAN_POINT('Ctrl Pts',(-88.0629053119781,-7.75898237652218,
9.33006918526815));
#35821=CARTESIAN_POINT('Ctrl Pts',(-87.9435504073892,-11.2820095247355,
4.46858586391342));
#35822=CARTESIAN_POINT('Ctrl Pts',(-87.8241955028005,-12.0433194102992,
-1.48676027669951));
#35823=CARTESIAN_POINT('Ctrl Pts',(-87.7048405982117,-9.85655138039453,
-7.07816313888748));
#35824=CARTESIAN_POINT('Ctrl Pts',(-87.5854856936229,-5.25700324774061,
-10.9369061160659));
#35825=CARTESIAN_POINT('Ctrl Pts',(-87.4661307890341,0.629403984779391,
-12.1184095144703));
#35826=CARTESIAN_POINT('Ctrl Pts',(-87.3467758844454,6.36173974212238,-10.3334537300374));
#35827=CARTESIAN_POINT('Ctrl Pts',(-87.2274209798566,10.5367885258817,-6.01897716376213));
#35828=CARTESIAN_POINT('Ctrl Pts',(-87.1080660752678,12.1325423085809,-0.231118297790334));
#35829=CARTESIAN_POINT('Ctrl Pts',(-86.988711170679,10.7583773489877,5.61331589650015));
#35830=CARTESIAN_POINT('Ctrl Pts',(-86.8693562660902,6.75067477520012,10.0836694023829));
#35831=CARTESIAN_POINT('Ctrl Pts',(-86.7500013615015,1.09047802269313,12.085646702561));
#35832=CARTESIAN_POINT('Ctrl Pts',(-86.6306464569127,-4.83665627969321,
11.1291848115301));
#35833=CARTESIAN_POINT('Ctrl Pts',(-86.5112915523239,-9.57982799866117,
7.44841553977487));
#35834=CARTESIAN_POINT('Ctrl Pts',(-86.3919366477351,-11.9779585879509,
1.94435248924289));
#35835=CARTESIAN_POINT('Ctrl Pts',(-86.2725817431463,-11.4440109037837,
-4.03566759919234));
#35836=CARTESIAN_POINT('Ctrl Pts',(-86.1532268385576,-8.10868972297233,
-9.02779870808241));
#35837=CARTESIAN_POINT('Ctrl Pts',(-86.0338719339688,-2.78844658836103,
-11.8100196511669));
#35838=CARTESIAN_POINT('Ctrl Pts',(-85.91451702938,3.21437894110451,-11.7012720060716));
#35839=CARTESIAN_POINT('Ctrl Pts',(-85.7951621247913,8.43035831588801,-8.72817605246533));
#35840=CARTESIAN_POINT('Ctrl Pts',(-85.6758072202024,11.5826746487625,-3.61851440759975));
#35841=CARTESIAN_POINT('Ctrl Pts',(-85.5564523156137,11.8996740587416,2.37692150329029));
#35842=CARTESIAN_POINT('Ctrl Pts',(-85.4370974110249,9.30375842458687,7.79051203156894));
#35843=CARTESIAN_POINT('Ctrl Pts',(-85.317742506436,4.43038058867899,11.2970671581852));
#35844=CARTESIAN_POINT('Ctrl Pts',(-85.1983876018474,-1.52750781485411,
12.0382190714678));
#35845=CARTESIAN_POINT('Ctrl Pts',(-85.0790326972585,-7.11147837223829,
9.83254157877195));
#35846=CARTESIAN_POINT('Ctrl Pts',(-84.9596777926698,-10.9546338254212,
5.21996133012747));
#35847=CARTESIAN_POINT('Ctrl Pts',(-84.8403228880809,-12.1162101432834,
-0.670410546528588));
#35848=CARTESIAN_POINT('Ctrl Pts',(-84.7209679834922,-10.311865661126,-6.3966729730357));
#35849=CARTESIAN_POINT('Ctrl Pts',(-84.6016130789034,-5.98328492938166,
-10.5570971384632));
#35850=CARTESIAN_POINT('Ctrl Pts',(-84.4822581743146,-0.190058981459703,
-12.1332549680886));
#35851=CARTESIAN_POINT('Ctrl Pts',(-84.3629032697258,5.64969140599582,-10.7393196038696));
#35852=CARTESIAN_POINT('Ctrl Pts',(-84.243548365137,10.1064567629635,-6.71651176100154));
#35853=CARTESIAN_POINT('Ctrl Pts',(-84.1241934605483,12.0892678079849,-1.04957248595764));
#35854=CARTESIAN_POINT('Ctrl Pts',(-84.0048385559594,11.1127532533934,4.8742910938504));
#35855=CARTESIAN_POINT('Ctrl Pts',(-83.8854836513707,7.41595359043792,9.60497948355609));
#35856=CARTESIAN_POINT('Ctrl Pts',(-83.7661287467819,1.90380649294891,11.9844699247096));
#35857=CARTESIAN_POINT('Ctrl Pts',(-83.6467738421932,-4.07437241005299,
11.4302881855003));
#35858=CARTESIAN_POINT('Ctrl Pts',(-83.5274189376044,-9.05518780079726,
8.07809212706594));
#35859=CARTESIAN_POINT('Ctrl Pts',(-83.4080640330156,-11.8193884683451,
2.74846408379857));
#35860=CARTESIAN_POINT('Ctrl Pts',(-83.2887091284268,-11.6903271506389,
-3.25395905635905));
#35861=CARTESIAN_POINT('Ctrl Pts',(-83.169354223838,-8.69959672896538,-8.45984724884512));
#35862=CARTESIAN_POINT('Ctrl Pts',(-83.0499993192493,-3.57929649423348,
-11.5948538127748));
#35863=CARTESIAN_POINT('Ctrl Pts',(-82.9306444146604,2.41717779161743,-11.8915621351014));
#35864=CARTESIAN_POINT('Ctrl Pts',(-82.8112895100718,7.82195254969964,-9.27734110083463));
#35865=CARTESIAN_POINT('Ctrl Pts',(-82.6919346054828,11.3119952432111,-4.39212460189635));
#35866=CARTESIAN_POINT('Ctrl Pts',(-82.5725797008941,12.032981222132,1.56823791386042));
#35867=CARTESIAN_POINT('Ctrl Pts',(-82.4532247963053,9.80841843472616,7.14471205023903));
#35868=CARTESIAN_POINT('Ctrl Pts',(-82.3338698917165,5.18286116302566,10.9722363124425));
#35869=CARTESIAN_POINT('Ctrl Pts',(-82.2145149871278,-0.711412610965203,
12.1138715285492));
#35870=CARTESIAN_POINT('Ctrl Pts',(-82.095160082539,-6.43152634087976,10.2901605048943));
#35871=CARTESIAN_POINT('Ctrl Pts',(-81.9758051779502,-10.5772985709532,
5.94752208025603));
#35872=CARTESIAN_POINT('Ctrl Pts',(-81.8564502733614,-12.1338001704439,
0.149001836180137));
#35873=CARTESIAN_POINT('Ctrl Pts',(-81.7370953687727,-10.7201981070584,
-5.68601122528114));
#35874=CARTESIAN_POINT('Ctrl Pts',(-81.6177404641839,-6.68214906904267,
-10.1291094532373));
#35875=CARTESIAN_POINT('Ctrl Pts',(-81.4983855595951,-1.00891489896113,
-12.0927868699637));
#35876=CARTESIAN_POINT('Ctrl Pts',(-81.3790306550063,4.91237722573152,-11.0960912178675));
#35877=CARTESIAN_POINT('Ctrl Pts',(-81.2994607186138,8.05617789784086,-8.62079961508711));
#35878=CARTESIAN_POINT('Ctrl Pts',(-81.2596757504175,9.23632576486131,-7.08155775150208));
#35879=CARTESIAN_POINT('Ctrl Pts',(-90.1653242495824,6.59052307073355,-9.24336091171003));
#35880=CARTESIAN_POINT('Ctrl Pts',(-90.1255392813862,8.13093734776757,-8.14504440884377));
#35881=CARTESIAN_POINT('Ctrl Pts',(-90.0459693449936,10.6502898834801,-5.16422596603819));
#35882=CARTESIAN_POINT('Ctrl Pts',(-89.9266144404049,11.8223099934421,0.574166021916792));
#35883=CARTESIAN_POINT('Ctrl Pts',(-89.807259535816,10.100134848291,6.17095566716168));
#35884=CARTESIAN_POINT('Ctrl Pts',(-89.6879046312274,5.90564768780508,10.257678817313));
#35885=CARTESIAN_POINT('Ctrl Pts',(-89.5685497266385,0.265473343179258,
11.8331826029404));
#35886=CARTESIAN_POINT('Ctrl Pts',(-89.4491948220497,-5.43966365714846,
10.5121670117828));
#35887=CARTESIAN_POINT('Ctrl Pts',(-89.329839917461,-9.81323901452016,6.61782610743594));
#35888=CARTESIAN_POINT('Ctrl Pts',(-89.2104850128722,-11.7846314800909,
1.10353861496494));
#35889=CARTESIAN_POINT('Ctrl Pts',(-89.0911301082834,-10.8712726183956,
-4.68089682639964));
#35890=CARTESIAN_POINT('Ctrl Pts',(-88.9717752036946,-7.29673936272674,
-9.31949155569622));
#35891=CARTESIAN_POINT('Ctrl Pts',(-88.8524202991058,-1.93604164128715,
-11.6767758614481));
#35892=CARTESIAN_POINT('Ctrl Pts',(-88.7330653945171,3.89857898923652,-11.175706772923));
#35893=CARTESIAN_POINT('Ctrl Pts',(-88.6137104899282,8.7788683554999,-7.9389429314306));
#35894=CARTESIAN_POINT('Ctrl Pts',(-88.4943555853395,11.5101831526637,-2.7588090212386));
#35895=CARTESIAN_POINT('Ctrl Pts',(-88.3750006807507,11.4239261515159,3.09665215350583));
#35896=CARTESIAN_POINT('Ctrl Pts',(-88.2556457761619,8.54121220482409,8.19408553260299));
#35897=CARTESIAN_POINT('Ctrl Pts',(-88.1362908715732,3.56769934299305,11.2856929235474));
#35898=CARTESIAN_POINT('Ctrl Pts',(-88.0169359669843,-2.27914878806212,
11.6146814126363));
#35899=CARTESIAN_POINT('Ctrl Pts',(-87.8975810623956,-7.56808527045601,
9.10051805079796));
#35900=CARTESIAN_POINT('Ctrl Pts',(-87.7782261578068,-11.00443408193,4.35864359723029));
#35901=CARTESIAN_POINT('Ctrl Pts',(-87.658871253218,-11.7470131794959,-1.45018096507549));
#35902=CARTESIAN_POINT('Ctrl Pts',(-87.5395163486293,-9.61404701023339,
-6.90401647971133));
#35903=CARTESIAN_POINT('Ctrl Pts',(-87.4201614440405,-5.12766325727862,
-10.6678213797489));
#35904=CARTESIAN_POINT('Ctrl Pts',(-87.3008065394517,0.613918526324883,
-11.8202558141297));
#35905=CARTESIAN_POINT('Ctrl Pts',(-87.1814516348629,6.20521951209942,-10.0792159554161));
#35906=CARTESIAN_POINT('Ctrl Pts',(-87.0620967302741,10.2775480302584,-5.87089004791594));
#35907=CARTESIAN_POINT('Ctrl Pts',(-86.9427418256853,11.8340408938926,-0.225432009039294));
#35908=CARTESIAN_POINT('Ctrl Pts',(-86.8233869210966,10.4936850217949,5.47520941448009));
#35909=CARTESIAN_POINT('Ctrl Pts',(-86.7040320165078,6.58458543306176,9.83557716373216));
#35910=CARTESIAN_POINT('Ctrl Pts',(-86.584677111919,1.06364858957175,11.7882990777696));
#35911=CARTESIAN_POINT('Ctrl Pts',(-86.4653222073302,-4.71765824077202,
10.8553693715279));
#35912=CARTESIAN_POINT('Ctrl Pts',(-86.3459673027413,-9.3441319559572,7.26515942417602));
#35913=CARTESIAN_POINT('Ctrl Pts',(-86.2266123981528,-11.6832604535745,
1.89651486758619));
#35914=CARTESIAN_POINT('Ctrl Pts',(-86.1072574935638,-11.1624496812795,
-3.93637658030022));
#35915=CARTESIAN_POINT('Ctrl Pts',(-85.9879025889751,-7.90918863803782,
-8.80568444568433));
#35916=CARTESIAN_POINT('Ctrl Pts',(-85.8685476843863,-2.71984140815738,
-11.5194533804129));
#35917=CARTESIAN_POINT('Ctrl Pts',(-85.7491927797975,3.13529439007966,-11.413381293752));
#35918=CARTESIAN_POINT('Ctrl Pts',(-85.6298378752087,8.2229430998832,-8.51343351680839));
#35919=CARTESIAN_POINT('Ctrl Pts',(-85.51048297062,11.2977018309809,-3.52948676258799));
#35920=CARTESIAN_POINT('Ctrl Pts',(-85.3911280660312,11.6069019875202,2.31844122658576));
#35921=CARTESIAN_POINT('Ctrl Pts',(-85.2717731614424,9.07485462346901,7.59883918976686));
#35922=CARTESIAN_POINT('Ctrl Pts',(-85.1524182568537,4.32137830047819,11.0191212468685));
#35923=CARTESIAN_POINT('Ctrl Pts',(-85.0330633522648,-1.48992597651517,
11.7420383261825));
#35924=CARTESIAN_POINT('Ctrl Pts',(-84.9137084476761,-6.93651204608445,
9.59062793061848));
#35925=CARTESIAN_POINT('Ctrl Pts',(-84.7943535430873,-10.6851129277304,
5.09153269563102));
#35926=CARTESIAN_POINT('Ctrl Pts',(-84.6749986384985,-11.8181105548836,
-0.653916188506099));
#35927=CARTESIAN_POINT('Ctrl Pts',(-84.5556437339097,-10.058159025729,-6.23929326784405));
#35928=CARTESIAN_POINT('Ctrl Pts',(-84.436288829321,-5.83607596274649,-10.2973569825517));
#35929=CARTESIAN_POINT('Ctrl Pts',(-84.3169339247321,-0.185382890217079,
-11.8347360195755));
#35930=CARTESIAN_POINT('Ctrl Pts',(-84.1975790201434,5.510689963895,-10.4750961614113));
#35931=CARTESIAN_POINT('Ctrl Pts',(-84.0782241155545,9.85780387847308,-6.55126294410587));
#35932=CARTESIAN_POINT('Ctrl Pts',(-83.9588692109658,11.7918310918008,-1.02374946684855));
#35933=CARTESIAN_POINT('Ctrl Pts',(-83.839514306377,10.8393420850784,4.75436711171122));
#35934=CARTESIAN_POINT('Ctrl Pts',(-83.7201594017883,7.23349614815536,9.36866462958968));
#35935=CARTESIAN_POINT('Ctrl Pts',(-83.6008044971995,1.85696643939838,11.6896115895125));
#35936=CARTESIAN_POINT('Ctrl Pts',(-83.4814495926107,-3.97412912241924,
11.149064588097));
#35937=CARTESIAN_POINT('Ctrl Pts',(-83.3620946880219,-8.83239967444598,
7.87934384607241));
#35938=CARTESIAN_POINT('Ctrl Pts',(-83.2427397834332,-11.5285916931254,
2.68084260790612));
#35939=CARTESIAN_POINT('Ctrl Pts',(-83.1233848788443,-11.4027057186355,
-3.17390070115562));
#35940=CARTESIAN_POINT('Ctrl Pts',(-83.0040299742556,-8.48555734094881,
-8.25170650574289));
#35941=CARTESIAN_POINT('Ctrl Pts',(-82.8846750696667,-3.49123374201361,
-11.3095813465276));
#35942=CARTESIAN_POINT('Ctrl Pts',(-82.765320165078,2.35770707459874,-11.5989896445302));
#35943=CARTESIAN_POINT('Ctrl Pts',(-82.6459652604892,7.6295061652301,-9.04908725487964));
#35944=CARTESIAN_POINT('Ctrl Pts',(-82.5266103559004,11.0336820507108,-4.28406353985282));
#35945=CARTESIAN_POINT('Ctrl Pts',(-82.4072554513116,11.7369293455864,1.52965397786838));
#35946=CARTESIAN_POINT('Ctrl Pts',(-82.2879005467229,9.56709829718583,6.96892806364386));
#35947=CARTESIAN_POINT('Ctrl Pts',(-82.1685456421341,5.05534531762843,10.7022823342691));
#35948=CARTESIAN_POINT('Ctrl Pts',(-82.0491907375453,-0.69390946402377,
11.8158294779506));
#35949=CARTESIAN_POINT('Ctrl Pts',(-81.9298358329566,-6.27328912541999,
10.0369878894641));
#35950=CARTESIAN_POINT('Ctrl Pts',(-81.8104809283677,-10.3170613917449,
5.8011930001925));
#35951=CARTESIAN_POINT('Ctrl Pts',(-81.691126023779,-11.8352678081161,0.145335889030752));
#35952=CARTESIAN_POINT('Ctrl Pts',(-81.5717711191901,-10.4564451178409,
-5.54611619326633));
#35953=CARTESIAN_POINT('Ctrl Pts',(-81.4524162146015,-6.5177456901353,-9.87989923625037));
#35954=CARTESIAN_POINT('Ctrl Pts',(-81.3330613100126,-0.984092193465425,
-11.7952635729993));
#35955=CARTESIAN_POINT('Ctrl Pts',(-81.2137064054239,4.79151619643789,-10.82308999176));
#35956=CARTESIAN_POINT('Ctrl Pts',(-81.1341364690313,7.85796878071416,-8.40869890153527));
#35957=CARTESIAN_POINT('Ctrl Pts',(-81.0943515008351,9.00908103434978,-6.90732757341935));
#35958=CARTESIAN_POINT('Ctrl Pts',(-90.,6.42428395783973,-9.01020671414053));
#35959=CARTESIAN_POINT('Ctrl Pts',(-89.9602150318037,7.92584288148909,-7.93959410657265));
#35960=CARTESIAN_POINT('Ctrl Pts',(-89.8806450954112,10.3816473609839,-5.03396371914769));
#35961=CARTESIAN_POINT('Ctrl Pts',(-89.7612901908224,11.5241044785577,0.559683279179561));
#35962=CARTESIAN_POINT('Ctrl Pts',(-89.6419352862336,9.84536941628095,6.01529970711026));
#35963=CARTESIAN_POINT('Ctrl Pts',(-89.5225803816449,5.75668384652155,9.99893950199032));
#35964=CARTESIAN_POINT('Ctrl Pts',(-89.4032254770561,0.258777053280351,
11.5347028377517));
#35965=CARTESIAN_POINT('Ctrl Pts',(-89.2838705724674,-5.30245378001128,
10.2470084955505));
#35966=CARTESIAN_POINT('Ctrl Pts',(-89.1645156678784,-9.56571023252816,
6.45089830374292));
#35967=CARTESIAN_POINT('Ctrl Pts',(-89.0451607632898,-11.4873763666492,
1.07570299730198));
#35968=CARTESIAN_POINT('Ctrl Pts',(-88.925805858701,-10.5970560354761,-4.56282605605006));
#35969=CARTESIAN_POINT('Ctrl Pts',(-88.8064509541122,-7.11268667591289,
-9.08441704154723));
#35970=CARTESIAN_POINT('Ctrl Pts',(-88.6870960495234,-1.88720699773628,
-11.3822412941864));
#35971=CARTESIAN_POINT('Ctrl Pts',(-88.5677411449346,3.80024137539898,-10.8938111540241));
#35972=CARTESIAN_POINT('Ctrl Pts',(-88.4483862403457,8.55743050117986,-7.73869132528777));
#35973=CARTESIAN_POINT('Ctrl Pts',(-88.3290313357571,11.2198507137954,-2.6892209233878));
#35974=CARTESIAN_POINT('Ctrl Pts',(-88.2096764311682,11.1357694560897,3.01854231284303));
#35975=CARTESIAN_POINT('Ctrl Pts',(-88.0903215265796,8.32576898055664,7.9873982188198));
#35976=CARTESIAN_POINT('Ctrl Pts',(-87.9709666219907,3.47770782525073,11.0010230180077));
#35977=CARTESIAN_POINT('Ctrl Pts',(-87.8516117174019,-2.22165962238982,
11.3217131134804));
#35978=CARTESIAN_POINT('Ctrl Pts',(-87.7322568128132,-7.37718816438983,
8.87096691632776));
#35979=CARTESIAN_POINT('Ctrl Pts',(-87.6129019082243,-10.7268586391246,
4.24870133054717));
#35980=CARTESIAN_POINT('Ctrl Pts',(-87.4935470036356,-11.4507069486926,
-1.41360165345147));
#35981=CARTESIAN_POINT('Ctrl Pts',(-87.3741920990468,-9.37154264007224,
-6.72986982053519));
#35982=CARTESIAN_POINT('Ctrl Pts',(-87.2548371944581,-4.99832326681662,
-10.398736643432));
#35983=CARTESIAN_POINT('Ctrl Pts',(-87.1354822898692,0.598433067870375,
-11.5221021137892));
#35984=CARTESIAN_POINT('Ctrl Pts',(-87.0161273852805,6.04869928207646,-9.82497818079478));
#35985=CARTESIAN_POINT('Ctrl Pts',(-86.8967724806917,10.0183075346351,-5.72280293206974));
#35986=CARTESIAN_POINT('Ctrl Pts',(-86.7774175761028,11.5355394792043,-0.219745720288259));
#35987=CARTESIAN_POINT('Ctrl Pts',(-86.6580626715142,10.2289926946021,5.33710293246003));
#35988=CARTESIAN_POINT('Ctrl Pts',(-86.5387077669253,6.41849609092341,9.58748492508142));
#35989=CARTESIAN_POINT('Ctrl Pts',(-86.4193528623365,1.03681915645036,11.4909514529782));
#35990=CARTESIAN_POINT('Ctrl Pts',(-86.2999979577478,-4.59866020185083,
10.5815539315257));
#35991=CARTESIAN_POINT('Ctrl Pts',(-86.1806430531589,-9.10843591325322,
7.08190330857717));
#35992=CARTESIAN_POINT('Ctrl Pts',(-86.0612881485703,-11.3885623191981,
1.8486772459295));
#35993=CARTESIAN_POINT('Ctrl Pts',(-85.9419332439815,-10.8808884587753,
-3.83708556140811));
#35994=CARTESIAN_POINT('Ctrl Pts',(-85.8225783393926,-7.7096875531033,-8.58357018328625));
#35995=CARTESIAN_POINT('Ctrl Pts',(-85.7032234348039,-2.65123622795373,
-11.2288871096588));
#35996=CARTESIAN_POINT('Ctrl Pts',(-85.583868530215,3.05620983905482,-11.1254905814324));
#35997=CARTESIAN_POINT('Ctrl Pts',(-85.4645136256263,8.01552788387837,-8.29869098115147));
#35998=CARTESIAN_POINT('Ctrl Pts',(-85.3451587210375,11.0127290131994,-3.44045911757623));
#35999=CARTESIAN_POINT('Ctrl Pts',(-85.2258038164487,11.3141299162988,2.25996094988123));
#36000=CARTESIAN_POINT('Ctrl Pts',(-85.10644891186,8.84595082235115,7.40716634796478));
#36001=CARTESIAN_POINT('Ctrl Pts',(-84.9870940072712,4.21237601227739,10.7411753355518));
#36002=CARTESIAN_POINT('Ctrl Pts',(-84.8677391026824,-1.45234413817624,
11.4458575808972));
#36003=CARTESIAN_POINT('Ctrl Pts',(-84.7483841980936,-6.7615457199306,9.34871428246502));
#36004=CARTESIAN_POINT('Ctrl Pts',(-84.6290292935049,-10.4155920300395,
4.96310406113458));
#36005=CARTESIAN_POINT('Ctrl Pts',(-84.509674388916,-11.5200109664838,-0.637421830483606));
#36006=CARTESIAN_POINT('Ctrl Pts',(-84.3903194843273,-9.80445239033203,
-6.08191356265241));
#36007=CARTESIAN_POINT('Ctrl Pts',(-84.2709645797384,-5.68886699611132,
-10.0376168266402));
#36008=CARTESIAN_POINT('Ctrl Pts',(-84.1516096751498,-0.180706798974452,
-11.5362170710623));
#36009=CARTESIAN_POINT('Ctrl Pts',(-84.0322547705609,5.37168852179416,-10.2108727189529));
#36010=CARTESIAN_POINT('Ctrl Pts',(-83.9128998659722,9.60915099398264,-6.38601412721019));
#36011=CARTESIAN_POINT('Ctrl Pts',(-83.7935449613833,11.4943943756167,-0.99792644773947));
#36012=CARTESIAN_POINT('Ctrl Pts',(-83.6741900567946,10.5659309167634,4.63444312957206));
#36013=CARTESIAN_POINT('Ctrl Pts',(-83.5548351522057,7.0510387058728,9.13234977562325));
#36014=CARTESIAN_POINT('Ctrl Pts',(-83.4354802476171,1.81012638584784,11.3947532543155));
#36015=CARTESIAN_POINT('Ctrl Pts',(-83.3161253430282,-3.87388583478548,
10.8678409906937));
#36016=CARTESIAN_POINT('Ctrl Pts',(-83.1967704384395,-8.6096115480947,7.68059556507888));
#36017=CARTESIAN_POINT('Ctrl Pts',(-83.0774155338507,-11.2377949179057,
2.61322113201366));
#36018=CARTESIAN_POINT('Ctrl Pts',(-82.9580606292619,-11.1150842866322,
-3.09384234595218));
#36019=CARTESIAN_POINT('Ctrl Pts',(-82.8387057246731,-8.27151795293221,
-8.04356576264067));
#36020=CARTESIAN_POINT('Ctrl Pts',(-82.7193508200843,-3.40317098979375,
-11.0243088802804));
#36021=CARTESIAN_POINT('Ctrl Pts',(-82.5999959154955,2.29823635758004,-11.306417153959));
#36022=CARTESIAN_POINT('Ctrl Pts',(-82.4806410109068,7.43705978076056,-8.82083340892465));
#36023=CARTESIAN_POINT('Ctrl Pts',(-82.361286106318,10.7553688582105,-4.17600247780928));
#36024=CARTESIAN_POINT('Ctrl Pts',(-82.2419312017292,11.4408774690408,1.49107004187632));
#36025=CARTESIAN_POINT('Ctrl Pts',(-82.1225762971404,9.32577815964549,6.79314407704868));
#36026=CARTESIAN_POINT('Ctrl Pts',(-82.0032213925517,4.92782947223121,10.4323283560957));
#36027=CARTESIAN_POINT('Ctrl Pts',(-81.8838664879629,-0.676406317082347,
11.5177874273519));
#36028=CARTESIAN_POINT('Ctrl Pts',(-81.7645115833741,-6.1150519099602,9.78381527403391));
#36029=CARTESIAN_POINT('Ctrl Pts',(-81.6451566787853,-10.0568242125366,
5.65486392012898));
#36030=CARTESIAN_POINT('Ctrl Pts',(-81.5258017741966,-11.5367354457883,
0.14166994188137));
#36031=CARTESIAN_POINT('Ctrl Pts',(-81.4064468696077,-10.1926921286234,
-5.40622116125151));
#36032=CARTESIAN_POINT('Ctrl Pts',(-81.287091965019,-6.35334231122792,-9.63068901926348));
#36033=CARTESIAN_POINT('Ctrl Pts',(-81.1677370604302,-0.959269487969727,
-11.497740276035));
#36034=CARTESIAN_POINT('Ctrl Pts',(-81.0483821558414,4.67065516714427,-10.5500887656525));
#36035=CARTESIAN_POINT('Ctrl Pts',(-80.9688122194489,7.65975966358745,-8.19659818798342));
#36036=CARTESIAN_POINT('Ctrl Pts',(-80.9290272512526,8.78183630383825,-6.73309739533661));
#36037=CARTESIAN_POINT('Ctrl Pts',(-81.425,9.46357049537263,-7.25578792958508));
#36038=CARTESIAN_POINT('Ctrl Pts',(-81.4647849681962,8.25438701496738,-8.8329003286391));
#36039=CARTESIAN_POINT('Ctrl Pts',(-81.5045699363925,6.64381263499625,-10.1009963863071));
#36040=CARTESIAN_POINT('Ctrl Pts',(-81.5443549045888,4.82736280176375,-10.9052473689665));
#36041=CARTESIAN_POINT('Ctrl Pts',(-81.584139872785,3.01091296853115,-11.7094983516261));
#36042=CARTESIAN_POINT('Ctrl Pts',(-81.6239248409813,0.988587682037159,
-12.049904259277));
#36043=CARTESIAN_POINT('Ctrl Pts',(-81.6637098091776,-0.991377435125372,
-11.8847754636519));
#36044=CARTESIAN_POINT('Ctrl Pts',(-81.7034947773738,-2.97134255228793,
-11.7196466680267));
#36045=CARTESIAN_POINT('Ctrl Pts',(-81.7432797455701,-4.90894750011903,
-11.0489831691254));
#36046=CARTESIAN_POINT('Ctrl Pts',(-81.7830647137663,-6.56731641542222,
-9.95491585085338));
#36047=CARTESIAN_POINT('Ctrl Pts',(-81.8228496819626,-8.22568533072536,
-8.86084853258138));
#36048=CARTESIAN_POINT('Ctrl Pts',(-81.8626346501588,-9.6048182135006,-7.34337739493867));
#36049=CARTESIAN_POINT('Ctrl Pts',(-81.9024196183551,-10.5357815609709,
-5.58821281934641));
#36050=CARTESIAN_POINT('Ctrl Pts',(-81.9412274631861,-11.4438803422434,
-3.87615528629842));
#36051=CARTESIAN_POINT('Ctrl Pts',(-81.9800353080171,-11.9255534427014,
-1.93793649480206));
#36052=CARTESIAN_POINT('Ctrl Pts',(-82.0188431528482,-11.9260172048445,
5.30405712340781E-5));
#36053=CARTESIAN_POINT('Origin',(-85.75,0.,0.));
#36054=CARTESIAN_POINT('Origin',(-81.425,0.,0.));
#36055=CARTESIAN_POINT('Origin',(-94.,-5.,-2.88675134594813));
#36056=CARTESIAN_POINT('',(-89.,-5.,-2.88675134594813));
#36057=CARTESIAN_POINT('',(-94.,-5.,-2.88675134594813));
#36058=CARTESIAN_POINT('',(-89.,-5.,-2.88675134594813));
#36059=CARTESIAN_POINT('Origin',(-94.,-5.,2.88675134594813));
#36060=CARTESIAN_POINT('',(-89.,-5.,2.88675134594813));
#36061=CARTESIAN_POINT('',(-94.,-5.,2.88675134594813));
#36062=CARTESIAN_POINT('',(-89.,-5.,2.88675134594813));
#36063=CARTESIAN_POINT('Origin',(-94.,3.53525079574969E-16,5.77350269189626));
#36064=CARTESIAN_POINT('',(-89.,3.53525079574969E-16,5.77350269189626));
#36065=CARTESIAN_POINT('Origin',(-89.,0.,0.));
#36066=CARTESIAN_POINT('Origin',(-81.25,0.,0.));
#36067=CARTESIAN_POINT('',(-81.,-11.5,-1.40834381901946E-15));
#36068=CARTESIAN_POINT('Origin',(-81.,0.,0.));
#36069=CARTESIAN_POINT('',(-81.25,-11.75,-1.43895998899814E-15));
#36070=CARTESIAN_POINT('Origin',(-81.,0.,0.));
#56607=UNCERTAINTY_MEASURE_WITH_UNIT(LENGTH_MEASURE(0.01),#56640,
'DISTANCE_ACCURACY_VALUE',
'Maximum model space distance between geometric entities at asserted c
onnectivities');
#56617=UNCERTAINTY_MEASURE_WITH_UNIT(LENGTH_MEASURE(0.01),#56640,
'DISTANCE_ACCURACY_VALUE',
'Maximum model space distance between geometric entities at asserted c
onnectivities');
#56629=(
GEOMETRIC_REPRESENTATION_CONTEXT(3)
GLOBAL_UNCERTAINTY_ASSIGNED_CONTEXT((#56607))
GLOBAL_UNIT_ASSIGNED_CONTEXT((#56640,#56642,#56643))
REPRESENTATION_CONTEXT('','3D')
);
#56639=(
GEOMETRIC_REPRESENTATION_CONTEXT(3)
GLOBAL_UNCERTAINTY_ASSIGNED_CONTEXT((#56617))
GLOBAL_UNIT_ASSIGNED_CONTEXT((#56640,#56642,#56643))
REPRESENTATION_CONTEXT('','3D')
);
#56640=(
LENGTH_UNIT()
NAMED_UNIT(*)
SI_UNIT(.MILLI.,.METRE.)
);
#56642=(
NAMED_UNIT(*)
PLANE_ANGLE_UNIT()
SI_UNIT($,.RADIAN.)
);
#56643=(
NAMED_UNIT(*)
SI_UNIT($,.STERADIAN.)
SOLID_ANGLE_UNIT()
);
#56655=SHAPE_DEFINITION_REPRESENTATION(#56676,#56755);
#56676=PRODUCT_DEFINITION_SHAPE('',$,#56777);
#56755=SHAPE_REPRESENTATION('',(#18010),#56629);
#56765=PRODUCT_DEFINITION_CONTEXT('part definition',#56830,'design');
#56777=PRODUCT_DEFINITION('2026-10-26-00-02-49-069',
'11_Manifold_End_Cap_M24x1.5',#56798,#56765);
#56798=PRODUCT_DEFINITION_FORMATION('',$,#56843);
#56830=APPLICATION_CONTEXT(
'Core Data for Automotive Mechanical Design Process');
#56831=PRODUCT_CONTEXT('part definition',#56830,'mechanical');
#56843=PRODUCT('2026-10-26-00-02-49-069','11_Manifold_End_Cap_M24x1.5',
$,(#56831));
#56895=COLOUR_RGB('Light Blue',0.38,0.62,0.78);
#56896=FILL_AREA_STYLE_COLOUR('',#56895);
#56897=FILL_AREA_STYLE('',(#56896));
#56898=SURFACE_STYLE_FILL_AREA(#56897);
#56899=SURFACE_SIDE_STYLE('',(#56898));
#56900=SURFACE_STYLE_USAGE(.BOTH.,#56899);
#56901=PRESENTATION_STYLE_ASSIGNMENT((#56900));
ENDSEC;
END-ISO-10303-21;
